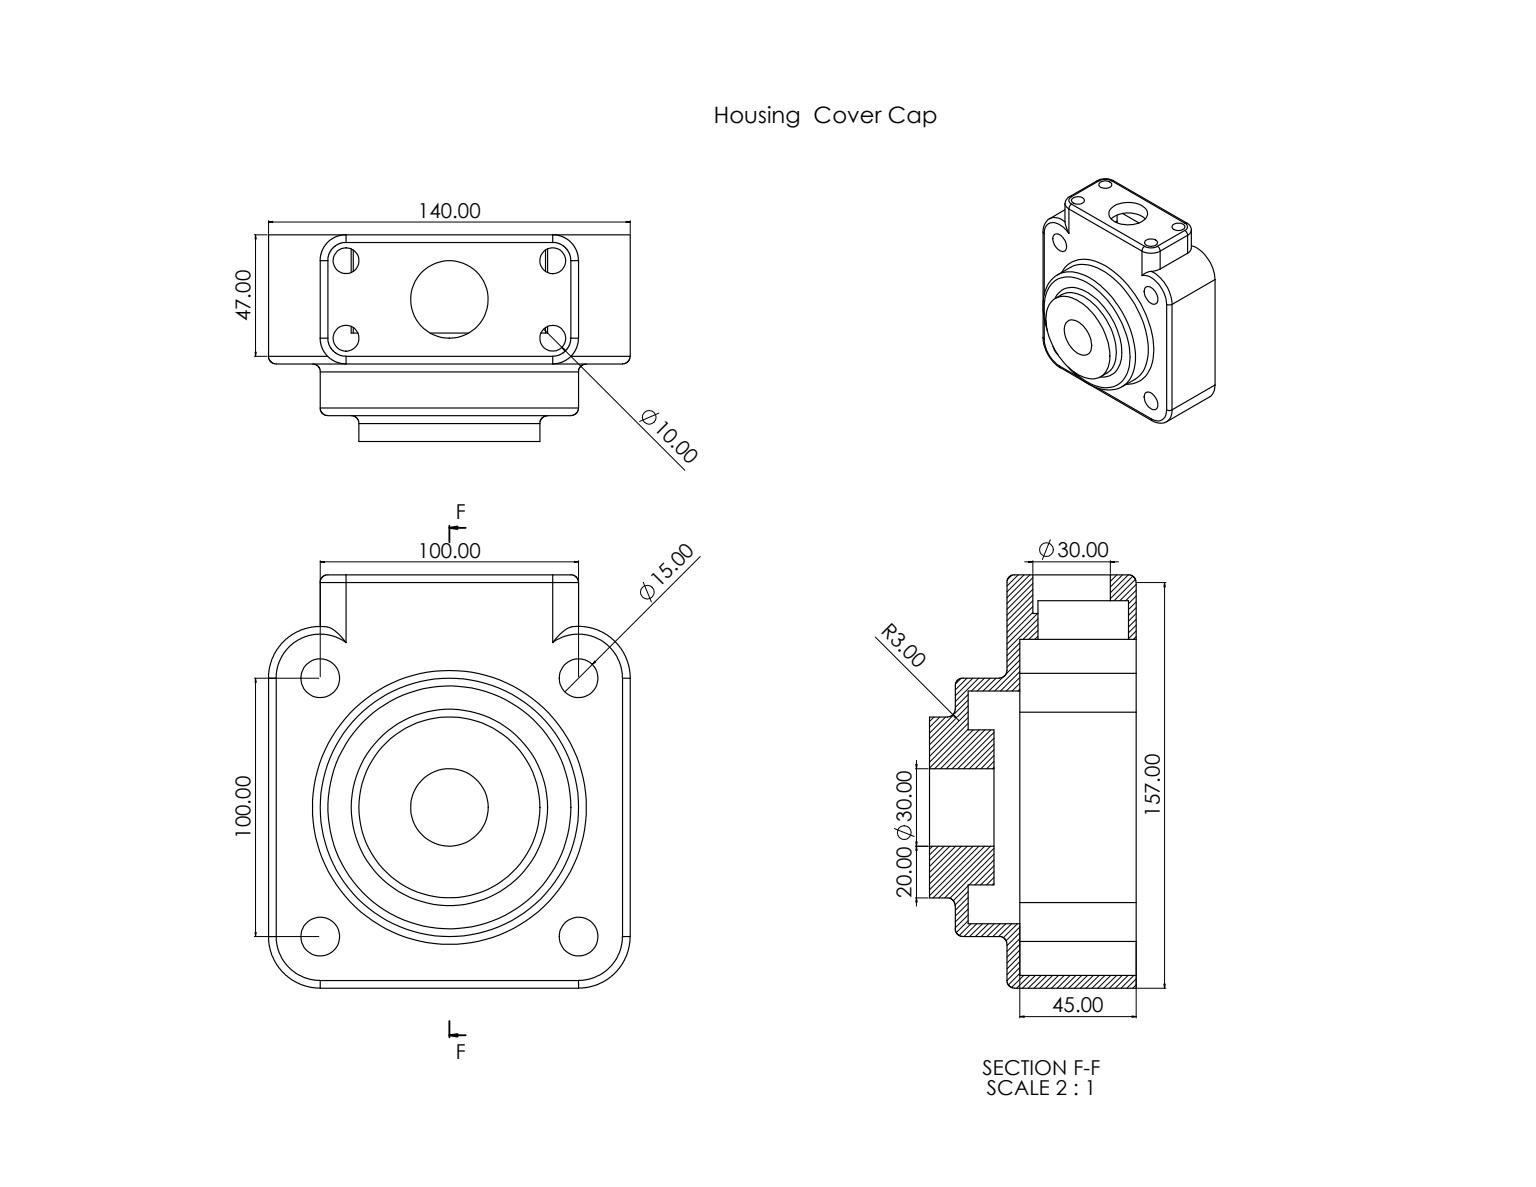
ISO-10303-21;
HEADER;
FILE_DESCRIPTION (('STEP AP214'),
    '1' );
FILE_NAME ('Housing  Cover Cap.step',
    '2026-10-18T20:16:25',
    ( '' ),
    ( '' ),
    'SwSTEP 2.0',
    'SolidWorks 2025',
    '' );
FILE_SCHEMA (( 'AUTOMOTIVE_DESIGN' ));
ENDSEC;

DATA;
#3=CARTESIAN_POINT ( 'NONE',  ( 37.16608720827707657, 51.86186943028246787, 12.49999999999999112 ) ) ;
#18=VERTEX_POINT ( 'NONE', #24496 ) ;
#21=CARTESIAN_POINT ( 'NONE',  ( -49.99999999999955236, -4.926614671774132148E-13, 82.49999999999998579 ) ) ;
#23=LINE ( 'NONE', #9535, #4037 ) ;
#27=ADVANCED_FACE ( 'NONE', ( #781 ), #12350, .T. ) ;
#31=DIRECTION ( 'NONE',  ( 0.000000000000000000, 0.000000000000000000, 1.000000000000000000 ) ) ;
#50=AXIS2_PLACEMENT_3D ( 'NONE', #18602, #5013, #4398 ) ;
#93=ORIENTED_EDGE ( 'NONE', *, *, #3486, .F. ) ;
#114=CARTESIAN_POINT ( 'NONE',  ( 57.49999999999998579, -50.00000000000000000, 97.07879600563551037 ) ) ;
#119=VERTEX_POINT ( 'NONE', #15443 ) ;
#124=AXIS2_PLACEMENT_3D ( 'NONE', #18042, #3695, #8540 ) ;
#129=ORIENTED_EDGE ( 'NONE', *, *, #25599, .F. ) ;
#146=ORIENTED_EDGE ( 'NONE', *, *, #2958, .F. ) ;
#148=CARTESIAN_POINT ( 'NONE',  ( -37.16608720827707657, -65.00000000000000000, 57.49999999999999289 ) ) ;
#164=DIRECTION ( 'NONE',  ( 1.000000000000000000, -0.000000000000000000, 0.000000000000000000 ) ) ;
#185=ORIENTED_EDGE ( 'NONE', *, *, #19570, .F. ) ;
#196=CARTESIAN_POINT ( 'NONE',  ( 39.99999999999998579, 87.00000000000001421, 12.49999999999999112 ) ) ;
#201=EDGE_CURVE ( 'NONE', #20672, #10252, #28885, .T. ) ;
#207=EDGE_CURVE ( 'NONE', #23407, #26039, #29815, .T. ) ;
#210=EDGE_CURVE ( 'NONE', #17431, #24948, #5944, .T. ) ;
#218=ORIENTED_EDGE ( 'NONE', *, *, #11268, .F. ) ;
#219=CARTESIAN_POINT ( 'NONE',  ( 50.00000000000045475, -4.865382331816764069E-13, 79.49999999999998579 ) ) ;
#228=VERTEX_POINT ( 'NONE', #15599 ) ;
#232=EDGE_CURVE ( 'NONE', #24670, #7391, #17304, .T. ) ;
#234=ADVANCED_FACE ( 'NONE', ( #15282 ), #1429, .T. ) ;
#238=EDGE_CURVE ( 'NONE', #14629, #10409, #29758, .T. ) ;
#241=EDGE_LOOP ( 'NONE', ( #4483, #26412, #12849, #13561 ) ) ;
#243=ADVANCED_FACE ( 'NONE', ( #23525 ), #20886, .F. ) ;
#270=ORIENTED_EDGE ( 'NONE', *, *, #22948, .T. ) ;
#284=ORIENTED_EDGE ( 'NONE', *, *, #16662, .T. ) ;
#291=PLANE ( 'NONE',  #12367 ) ;
#300=ORIENTED_EDGE ( 'NONE', *, *, #15085, .F. ) ;
#325=DIRECTION ( 'NONE',  ( 1.000000000000000000, 0.000000000000000000, 0.000000000000000000 ) ) ;
#327=DIRECTION ( 'NONE',  ( 1.000000000000000000, 0.000000000000000000, 0.000000000000000000 ) ) ;
#330=DIRECTION ( 'NONE',  ( 0.000000000000000000, 1.000000000000000000, -0.000000000000000000 ) ) ;
#340=CIRCLE ( 'NONE', #26766, 5.000000000000004441 ) ;
#346=VERTEX_POINT ( 'NONE', #26975 ) ;
#353=VERTEX_POINT ( 'NONE', #24142 ) ;
#375=DIRECTION ( 'NONE',  ( 0.000000000000000000, 0.000000000000000000, -1.000000000000000000 ) ) ;
#380=DIRECTION ( 'NONE',  ( 0.000000000000000000, 0.000000000000000000, 1.000000000000000000 ) ) ;
#381=EDGE_CURVE ( 'NONE', #9423, #9573, #2631, .T. ) ;
#390=CARTESIAN_POINT ( 'NONE',  ( 4.510281037539698445E-13, -4.926614671774132148E-13, 82.49999999999998579 ) ) ;
#392=ORIENTED_EDGE ( 'NONE', *, *, #26901, .T. ) ;
#395=EDGE_CURVE ( 'NONE', #119, #19467, #10261, .T. ) ;
#405=ORIENTED_EDGE ( 'NONE', *, *, #28102, .T. ) ;
#406=LINE ( 'NONE', #14743, #17330 ) ;
#412=EDGE_CURVE ( 'NONE', #8092, #2167, #25816, .T. ) ;
#422=ADVANCED_FACE ( 'NONE', ( #3565 ), #20954, .T. ) ;
#433=( LENGTH_UNIT ( ) NAMED_UNIT ( * ) SI_UNIT ( .MILLI., .METRE. ) );
#436=EDGE_CURVE ( 'NONE', #11277, #20672, #12935, .T. ) ;
#445=CARTESIAN_POINT ( 'NONE',  ( -50.00000000000000000, -50.00000000000000000, 97.07879600563551037 ) ) ;
#482=EDGE_CURVE ( 'NONE', #4513, #14016, #6055, .T. ) ;
#483=ADVANCED_FACE ( 'NONE', ( #14572 ), #23758, .T. ) ;
#498=VERTEX_POINT ( 'NONE', #7558 ) ;
#509=VERTEX_POINT ( 'NONE', #21581 ) ;
#528=FACE_OUTER_BOUND ( 'NONE', #3439, .T. ) ;
#532=AXIS2_PLACEMENT_3D ( 'NONE', #23516, #28832, #23662 ) ;
#535=EDGE_LOOP ( 'NONE', ( #1765, #22234, #5440, #4015 ) ) ;
#552=ADVANCED_FACE ( 'NONE', ( #7235 ), #23923, .F. ) ;
#569=ORIENTED_EDGE ( 'NONE', *, *, #16803, .T. ) ;
#628=CARTESIAN_POINT ( 'NONE',  ( -38.00000000000000711, 80.00000000000000000, 47.91742430504431383 ) ) ;
#634=AXIS2_PLACEMENT_3D ( 'NONE', #23126, #15969, #13490 ) ;
#640=DIRECTION ( 'NONE',  ( 1.000000000000000000, 0.000000000000000000, 4.565061778886335400E-17 ) ) ;
#648=CARTESIAN_POINT ( 'NONE',  ( -37.16608720827707657, 51.86186943028246787, 57.49999999999999289 ) ) ;
#655=AXIS2_PLACEMENT_3D ( 'NONE', #16975, #24609, #740 ) ;
#667=EDGE_LOOP ( 'NONE', ( #2923, #26532 ) ) ;
#671=DIRECTION ( 'NONE',  ( 0.000000000000000000, 0.000000000000000000, -1.000000000000000000 ) ) ;
#682=LINE ( 'NONE', #19245, #27844 ) ;
#702=FACE_OUTER_BOUND ( 'NONE', #5275, .T. ) ;
#707=PLANE ( 'NONE',  #25288 ) ;
#712=DIRECTION ( 'NONE',  ( 0.000000000000000000, -0.000000000000000000, 1.000000000000000000 ) ) ;
#719=DIRECTION ( 'NONE',  ( -1.000000000000000000, 1.224646799147308341E-16, 0.000000000000000000 ) ) ;
#731=PLANE ( 'NONE',  #2299 ) ;
#737=ORIENTED_EDGE ( 'NONE', *, *, #28020, .T. ) ;
#740=DIRECTION ( 'NONE',  ( 0.000000000000000000, 0.000000000000000000, -1.000000000000000000 ) ) ;
#747=ORIENTED_EDGE ( 'NONE', *, *, #23123, .T. ) ;
#754=AXIS2_PLACEMENT_3D ( 'NONE', #13903, #20910, #9218 ) ;
#756=DIRECTION ( 'NONE',  ( 0.000000000000000000, 0.000000000000000000, -1.000000000000000000 ) ) ;
#761=CARTESIAN_POINT ( 'NONE',  ( -67.00000000000000000, -50.00000000000000000, 62.49999999999999289 ) ) ;
#779=CARTESIAN_POINT ( 'NONE',  ( 49.75074519532149964, 69.99854282640310998, 54.74199497519533253 ) ) ;
#781=FACE_OUTER_BOUND ( 'NONE', #26889, .T. ) ;
#794=CARTESIAN_POINT ( 'NONE',  ( 46.83962869229247872, 69.75107682583961832, 59.80789731659786668 ) ) ;
#816=EDGE_LOOP ( 'NONE', ( #10122, #28506 ) ) ;
#817=ORIENTED_EDGE ( 'NONE', *, *, #19707, .F. ) ;
#822=CIRCLE ( 'NONE', #25229, 3.000000000000002665 ) ;
#833=CARTESIAN_POINT ( 'NONE',  ( -7.075845757273814415E-16, 65.00000000000000000, 15.49999999999998757 ) ) ;
#839=VECTOR ( 'NONE', #15202, 1000.000000000000000 ) ;
#847=ORIENTED_EDGE ( 'NONE', *, *, #7863, .T. ) ;
#854=DIRECTION ( 'NONE',  ( 1.000000000000000000, 0.000000000000000000, 0.000000000000000000 ) ) ;
#865=EDGE_CURVE ( 'NONE', #4126, #15180, #12302, .T. ) ;
#867=VECTOR ( 'NONE', #15137, 1000.000000000000000 ) ;
#869=DIRECTION ( 'NONE',  ( 0.000000000000000000, -0.000000000000000000, 1.000000000000000000 ) ) ;
#872=ORIENTED_EDGE ( 'NONE', *, *, #18796, .T. ) ;
#886=VERTEX_POINT ( 'NONE', #23419 ) ;
#921=ORIENTED_EDGE ( 'NONE', *, *, #28797, .F. ) ;
#932=LINE ( 'NONE', #24944, #23092 ) ;
#938=DIRECTION ( 'NONE',  ( -1.000000000000000000, 0.000000000000000000, 0.000000000000000000 ) ) ;
#941=AXIS2_PLACEMENT_3D ( 'NONE', #27026, #2189, #4376 ) ;
#945=DIRECTION ( 'NONE',  ( -1.000000000000000000, 0.000000000000000000, 0.000000000000000000 ) ) ;
#962=DIRECTION ( 'NONE',  ( 1.000000000000000000, 0.000000000000000000, 0.000000000000000000 ) ) ;
#963=VECTOR ( 'NONE', #30345, 1000.000000000000000 ) ;
#977=VERTEX_POINT ( 'NONE', #7367 ) ;
#980=CARTESIAN_POINT ( 'NONE',  ( 37.99999999999999289, 80.00000000000000000, 0.000000000000000000 ) ) ;
#987=ORIENTED_EDGE ( 'NONE', *, *, #11268, .T. ) ;
#996=DIRECTION ( 'NONE',  ( -1.000000000000000000, 0.000000000000000000, 0.000000000000000000 ) ) ;
#997=LINE ( 'NONE', #10507, #28045 ) ;
#1008=DIRECTION ( 'NONE',  ( 0.000000000000000000, 1.000000000000000000, -0.000000000000000000 ) ) ;
#1016=ORIENTED_EDGE ( 'NONE', *, *, #28061, .F. ) ;
#1019=LINE ( 'NONE', #10529, #11195 ) ;
#1024=LINE ( 'NONE', #9918, #9861 ) ;
#1030=CARTESIAN_POINT ( 'NONE',  ( 39.99999999999998579, 90.00000000000001421, 22.49999999999999289 ) ) ;
#1034=CARTESIAN_POINT ( 'NONE',  ( 39.99999999999998579, 90.00000000000001421, 52.49999999999999289 ) ) ;
#1043=CARTESIAN_POINT ( 'NONE',  ( -34.99999999999933920, 0.000000000000000000, 92.49999999999998579 ) ) ;
#1061=TOROIDAL_SURFACE ( 'NONE', #28508, 47.00000000000000000, 3.000000000000000000 ) ;
#1077=EDGE_LOOP ( 'NONE', ( #13664, #21788, #28119, #28909 ) ) ;
#1085=FACE_OUTER_BOUND ( 'NONE', #15743, .T. ) ;
#1094=VECTOR ( 'NONE', #9657, 1000.000000000000000 ) ;
#1114=DIRECTION ( 'NONE',  ( -1.000000000000000000, 0.000000000000000000, 0.000000000000000000 ) ) ;
#1118=ORIENTED_EDGE ( 'NONE', *, *, #29975, .T. ) ;
#1120=CARTESIAN_POINT ( 'NONE',  ( -41.02681369128806210, 65.11862996399604242, 62.46341648537969604 ) ) ;
#1132=AXIS2_PLACEMENT_3D ( 'NONE', #11394, #25726, #23672 ) ;
#1133=ORIENTED_EDGE ( 'NONE', *, *, #18687, .F. ) ;
#1151=AXIS2_PLACEMENT_3D ( 'NONE', #10819, #20330, #13767 ) ;
#1157=DIRECTION ( 'NONE',  ( -1.000000000000000000, 0.000000000000000000, 0.000000000000000000 ) ) ;
#1160=ORIENTED_EDGE ( 'NONE', *, *, #25599, .T. ) ;
#1161=DIRECTION ( 'NONE',  ( -0.000000000000000000, -0.000000000000000000, 1.000000000000000000 ) ) ;
#1189=CYLINDRICAL_SURFACE ( 'NONE', #21253, 10.00000000000000178 ) ;
#1215=ADVANCED_FACE ( 'NONE', ( #8102 ), #291, .T. ) ;
#1221=FACE_BOUND ( 'NONE', #816, .T. ) ;
#1222=VERTEX_POINT ( 'NONE', #12775 ) ;
#1225=ORIENTED_EDGE ( 'NONE', *, *, #15509, .T. ) ;
#1238=CARTESIAN_POINT ( 'NONE',  ( 0.000000000000000000, 0.000000000000000000, 82.49999999999998579 ) ) ;
#1243=CARTESIAN_POINT ( 'NONE',  ( 49.45745851869548204, 69.99439104891119712, 19.18218888609259665 ) ) ;
#1244=FACE_OUTER_BOUND ( 'NONE', #9042, .T. ) ;
#1252=LINE ( 'NONE', #3268, #8766 ) ;
#1257=ORIENTED_EDGE ( 'NONE', *, *, #26177, .F. ) ;
#1293=DIRECTION ( 'NONE',  ( 0.000000000000000000, -0.000000000000000000, -1.000000000000000000 ) ) ;
#1295=ORIENTED_EDGE ( 'NONE', *, *, #22144, .F. ) ;
#1301=AXIS2_PLACEMENT_3D ( 'NONE', #4447, #20953, #23150 ) ;
#1316=LINE ( 'NONE', #30013, #9536 ) ;
#1327=EDGE_CURVE ( 'NONE', #25485, #25063, #15100, .T. ) ;
#1349=LINE ( 'NONE', #8378, #16772 ) ;
#1356=DIRECTION ( 'NONE',  ( -1.000000000000000000, 0.000000000000000000, 0.000000000000000000 ) ) ;
#1365=EDGE_LOOP ( 'NONE', ( #17122, #18661, #20473, #30492 ) ) ;
#1369=AXIS2_PLACEMENT_3D ( 'NONE', #4710, #21541, #14681 ) ;
#1372=ORIENTED_EDGE ( 'NONE', *, *, #17855, .F. ) ;
#1376=VECTOR ( 'NONE', #15752, 1000.000000000000000 ) ;
#1403=CARTESIAN_POINT ( 'NONE',  ( 49.99999999999998579, 70.00000000000001421, 21.82070150977413903 ) ) ;
#1407=DIRECTION ( 'NONE',  ( 0.000000000000000000, 0.000000000000000000, 1.000000000000000000 ) ) ;
#1415=ORIENTED_EDGE ( 'NONE', *, *, #25806, .F. ) ;
#1418=EDGE_LOOP ( 'NONE', ( #23104, #19972, #12540, #30228 ) ) ;
#1423=ORIENTED_EDGE ( 'NONE', *, *, #5801, .F. ) ;
#1429=CYLINDRICAL_SURFACE ( 'NONE', #20294, 20.00000000000000355 ) ;
#1433=ORIENTED_EDGE ( 'NONE', *, *, #18979, .T. ) ;
#1440=FACE_BOUND ( 'NONE', #28403, .T. ) ;
#1442=CARTESIAN_POINT ( 'NONE',  ( 66.99999999999998579, 50.00000000000000000, 59.49999999999999289 ) ) ;
#1463=CARTESIAN_POINT ( 'NONE',  ( 66.99999999999998579, 50.00000000000000000, 62.49999999999999289 ) ) ;
#1468=AXIS2_PLACEMENT_3D ( 'NONE', #28004, #20963, #1806 ) ;
#1479=CARTESIAN_POINT ( 'NONE',  ( 49.99999999999998579, 50.00000000000000000, 12.49999999999999112 ) ) ;
#1515=CARTESIAN_POINT ( 'NONE',  ( 4.510281037539698445E-13, -4.926614671774132148E-13, 65.49999999999998579 ) ) ;
#1524=EDGE_CURVE ( 'NONE', #8240, #3050, #30833, .T. ) ;
#1528=CARTESIAN_POINT ( 'NONE',  ( -40.00000000000000000, 90.00000000000001421, 12.49999999999999112 ) ) ;
#1536=FACE_OUTER_BOUND ( 'NONE', #20558, .T. ) ;
#1548=CARTESIAN_POINT ( 'NONE',  ( 47.38379984956800683, 69.82936349420988620, 15.74781942413362401 ) ) ;
#1551=AXIS2_PLACEMENT_3D ( 'NONE', #27356, #5980, #30295 ) ;
#1572=EDGE_CURVE ( 'NONE', #27348, #886, #4923, .T. ) ;
#1577=ORIENTED_EDGE ( 'NONE', *, *, #1998, .F. ) ;
#1588=ORIENTED_EDGE ( 'NONE', *, *, #27343, .F. ) ;
#1589=CARTESIAN_POINT ( 'NONE',  ( 39.99999999999998579, 80.00000000000001421, 27.49999999999998934 ) ) ;
#1598=LINE ( 'NONE', #25900, #7425 ) ;
#1608=EDGE_CURVE ( 'NONE', #30496, #8380, #2142, .T. ) ;
#1616=CARTESIAN_POINT ( 'NONE',  ( 47.14142842854284510, 69.79466010243311302, 59.49999999999998579 ) ) ;
#1628=CARTESIAN_POINT ( 'NONE',  ( -38.00000000000000711, 65.00000000000000000, 50.49999999999998579 ) ) ;
#1646=FACE_OUTER_BOUND ( 'NONE', #22033, .T. ) ;
#1653=CARTESIAN_POINT ( 'NONE',  ( -47.82582523423074861, 69.88269270952190482, 16.26542374043941308 ) ) ;
#1663=DIRECTION ( 'NONE',  ( -1.000000000000000000, 0.000000000000000000, 0.000000000000000000 ) ) ;
#1684=VECTOR ( 'NONE', #5109, 1000.000000000000000 ) ;
#1688=VECTOR ( 'NONE', #24091, 1000.000000000000000 ) ;
#1696=ORIENTED_EDGE ( 'NONE', *, *, #28797, .T. ) ;
#1705=CIRCLE ( 'NONE', #23109, 3.000000000000002665 ) ;
#1714=CARTESIAN_POINT ( 'NONE',  ( -64.99999999999998579, -36.86186943028246787, 97.07879600563551037 ) ) ;
#1726=EDGE_LOOP ( 'NONE', ( #5104, #22705, #1867, #28955 ) ) ;
#1729=CARTESIAN_POINT ( 'NONE',  ( 39.99999999999998579, 90.00000000000001421, 59.49999999999999289 ) ) ;
#1736=LINE ( 'NONE', #23090, #25376 ) ;
#1747=ORIENTED_EDGE ( 'NONE', *, *, #14163, .F. ) ;
#1765=ORIENTED_EDGE ( 'NONE', *, *, #23091, .F. ) ;
#1771=ORIENTED_EDGE ( 'NONE', *, *, #28051, .F. ) ;
#1796=AXIS2_PLACEMENT_3D ( 'NONE', #16884, #14215, #26081 ) ;
#1799=FACE_OUTER_BOUND ( 'NONE', #1077, .T. ) ;
#1804=DIRECTION ( 'NONE',  ( 0.000000000000000000, 0.000000000000000000, 1.000000000000000000 ) ) ;
#1806=DIRECTION ( 'NONE',  ( 1.000000000000000000, 0.000000000000000000, 0.000000000000000000 ) ) ;
#1811=ORIENTED_EDGE ( 'NONE', *, *, #210, .F. ) ;
#1815=CARTESIAN_POINT ( 'NONE',  ( 53.00000000000045475, -4.861708391419322267E-13, 65.49999999999998579 ) ) ;
#1836=( NAMED_UNIT ( * ) PLANE_ANGLE_UNIT ( ) SI_UNIT ( $, .RADIAN. ) );
#1837=DIRECTION ( 'NONE',  ( -0.000000000000000000, 1.000000000000000000, -0.000000000000000000 ) ) ;
#1838=CARTESIAN_POINT ( 'NONE',  ( 39.99999999999998579, 80.00000000000001421, 17.49999999999999645 ) ) ;
#1841=AXIS2_PLACEMENT_3D ( 'NONE', #15376, #12910, #15536 ) ;
#1849=ORIENTED_EDGE ( 'NONE', *, *, #22349, .F. ) ;
#1857=DIRECTION ( 'NONE',  ( -0.000000000000000000, 1.000000000000000000, 0.000000000000000000 ) ) ;
#1861=ORIENTED_EDGE ( 'NONE', *, *, #16788, .T. ) ;
#1867=ORIENTED_EDGE ( 'NONE', *, *, #2489, .T. ) ;
#1868=AXIS2_PLACEMENT_3D ( 'NONE', #21433, #375, #22045 ) ;
#1892=AXIS2_PLACEMENT_3D ( 'NONE', #14281, #24110, #26306 ) ;
#1915=FACE_OUTER_BOUND ( 'NONE', #241, .T. ) ;
#1933=CARTESIAN_POINT ( 'NONE',  ( -15.00000000000004086, 1.571475800653548713E-14, 67.49999999999997158 ) ) ;
#1947=ADVANCED_FACE ( 'NONE', ( #3996 ), #10402, .F. ) ;
#1972=ADVANCED_FACE ( 'NONE', ( #14100 ), #16903, .F. ) ;
#1998=EDGE_CURVE ( 'NONE', #7862, #25485, #16458, .T. ) ;
#2013=ORIENTED_EDGE ( 'NONE', *, *, #27648, .F. ) ;
#2030=ORIENTED_EDGE ( 'NONE', *, *, #27366, .F. ) ;
#2037=DIRECTION ( 'NONE',  ( -1.000000000000000000, -0.000000000000000000, -0.000000000000000000 ) ) ;
#2056=ORIENTED_EDGE ( 'NONE', *, *, #20964, .F. ) ;
#2080=LINE ( 'NONE', #28140, #25328 ) ;
#2081=ORIENTED_EDGE ( 'NONE', *, *, #17855, .T. ) ;
#2085=CYLINDRICAL_SURFACE ( 'NONE', #8887, 29.99999999999928946 ) ;
#2088=CARTESIAN_POINT ( 'NONE',  ( 49.99999999999998579, 50.00000000000000000, 12.49999999999999112 ) ) ;
#2129=CARTESIAN_POINT ( 'NONE',  ( -57.50000000000001421, -50.00000000000000000, 12.49999999999999112 ) ) ;
#2133=( NAMED_UNIT ( * ) SI_UNIT ( $, .STERADIAN. ) SOLID_ANGLE_UNIT ( ) );
#2134=EDGE_CURVE ( 'NONE', #12801, #20802, #16920, .T. ) ;
#2138=ADVANCED_FACE ( 'NONE', ( #20141 ), #26435, .F. ) ;
#2142=LINE ( 'NONE', #2458, #29836 ) ;
#2150=CIRCLE ( 'NONE', #25556, 3.000000000000002665 ) ;
#2152=ADVANCED_FACE ( 'NONE', ( #24081 ), #22326, .T. ) ;
#2158=LINE ( 'NONE', #20876, #18238 ) ;
#2162=ORIENTED_EDGE ( 'NONE', *, *, #238, .F. ) ;
#2164=DIRECTION ( 'NONE',  ( 1.000000000000000000, 0.000000000000000000, 0.000000000000000000 ) ) ;
#2167=VERTEX_POINT ( 'NONE', #23767 ) ;
#2174=LINE ( 'NONE', #21178, #5076 ) ;
#2179=DIRECTION ( 'NONE',  ( -1.000000000000000000, 0.000000000000000000, 0.000000000000000000 ) ) ;
#2189=DIRECTION ( 'NONE',  ( 0.000000000000000000, 0.000000000000000000, -1.000000000000000000 ) ) ;
#2190=AXIS2_PLACEMENT_3D ( 'NONE', #7061, #2386, #6916 ) ;
#2198=ORIENTED_EDGE ( 'NONE', *, *, #12967, .F. ) ;
#2208=VECTOR ( 'NONE', #8117, 1000.000000000000000 ) ;
#2243=DIRECTION ( 'NONE',  ( 0.000000000000000000, 0.000000000000000000, 1.000000000000000000 ) ) ;
#2283=CIRCLE ( 'NONE', #19724, 15.00000000000000000 ) ;
#2299=AXIS2_PLACEMENT_3D ( 'NONE', #17276, #15551, #26809 ) ;
#2311=ORIENTED_EDGE ( 'NONE', *, *, #22140, .T. ) ;
#2313=VECTOR ( 'NONE', #14202, 1000.000000000000000 ) ;
#2317=DIRECTION ( 'NONE',  ( -0.000000000000000000, 1.000000000000000000, -0.000000000000000000 ) ) ;
#2324=ORIENTED_EDGE ( 'NONE', *, *, #18426, .T. ) ;
#2331=EDGE_LOOP ( 'NONE', ( #12248, #847, #22485, #24740 ) ) ;
#2373=ORIENTED_EDGE ( 'NONE', *, *, #8208, .T. ) ;
#2375=DIRECTION ( 'NONE',  ( -0.000000000000000000, -1.000000000000000000, -0.000000000000000000 ) ) ;
#2386=DIRECTION ( 'NONE',  ( 0.000000000000000000, 0.000000000000000000, 1.000000000000000000 ) ) ;
#2391=VECTOR ( 'NONE', #9153, 1000.000000000000000 ) ;
#2396=ORIENTED_EDGE ( 'NONE', *, *, #5540, .F. ) ;
#2399=ORIENTED_EDGE ( 'NONE', *, *, #24487, .T. ) ;
#2433=CIRCLE ( 'NONE', #26264, 29.99999999999928946 ) ;
#2449=CARTESIAN_POINT ( 'NONE',  ( 49.99999999999998579, -70.00000000000000000, 59.49999999999999289 ) ) ;
#2458=CARTESIAN_POINT ( 'NONE',  ( -52.16608720827707657, 36.86186943028246787, 97.07879600563551037 ) ) ;
#2479=ORIENTED_EDGE ( 'NONE', *, *, #16053, .F. ) ;
#2485=DIRECTION ( 'NONE',  ( -0.000000000000000000, -0.000000000000000000, 1.000000000000000000 ) ) ;
#2489=EDGE_CURVE ( 'NONE', #12801, #14860, #822, .T. ) ;
#2493=CARTESIAN_POINT ( 'NONE',  ( -34.99999999999933920, 0.000000000000000000, 92.49999999999998579 ) ) ;
#2498=EDGE_CURVE ( 'NONE', #28591, #119, #22243, .T. ) ;
#2520=ORIENTED_EDGE ( 'NONE', *, *, #6743, .F. ) ;
#2524=DIRECTION ( 'NONE',  ( 0.000000000000000000, 0.000000000000000000, 1.000000000000000000 ) ) ;
#2549=AXIS2_PLACEMENT_3D ( 'NONE', #12742, #10401, #25362 ) ;
#2550=DIRECTION ( 'NONE',  ( 1.000000000000000000, -0.000000000000000000, -0.000000000000000000 ) ) ;
#2558=ORIENTED_EDGE ( 'NONE', *, *, #18946, .F. ) ;
#2563=ADVANCED_FACE ( 'NONE', ( #12523 ), #16885, .F. ) ;
#2570=CARTESIAN_POINT ( 'NONE',  ( -50.00000000000000000, -50.00000000000000000, 97.07879600563551037 ) ) ;
#2571=VERTEX_POINT ( 'NONE', #18926 ) ;
#2574=CARTESIAN_POINT ( 'NONE',  ( 37.99999999999999289, 80.00000000000000000, 50.49999999999998579 ) ) ;
#2575=DIRECTION ( 'NONE',  ( 0.000000000000000000, 0.000000000000000000, 1.000000000000000000 ) ) ;
#2577=CARTESIAN_POINT ( 'NONE',  ( -40.00000000000002842, 80.00000000000001421, 22.49999999999983302 ) ) ;
#2583=DIRECTION ( 'NONE',  ( 0.000000000000000000, 0.000000000000000000, -1.000000000000000000 ) ) ;
#2600=ORIENTED_EDGE ( 'NONE', *, *, #27155, .F. ) ;
#2615=CARTESIAN_POINT ( 'NONE',  ( -50.00000000000000000, 70.00000000000000000, 52.49999999999999289 ) ) ;
#2620=ORIENTED_EDGE ( 'NONE', *, *, #14985, .F. ) ;
#2627=VERTEX_POINT ( 'NONE', #26083 ) ;
#2631=LINE ( 'NONE', #2790, #8152 ) ;
#2646=DIRECTION ( 'NONE',  ( -1.000000000000000000, 0.000000000000000000, 0.000000000000000000 ) ) ;
#2652=DIRECTION ( 'NONE',  ( -1.000000000000000000, 0.000000000000000000, 0.000000000000000000 ) ) ;
#2669=CARTESIAN_POINT ( 'NONE',  ( 47.14142842854284510, 69.79466010243311302, 59.49999999999998579 ) ) ;
#2683=EDGE_CURVE ( 'NONE', #27986, #27603, #13292, .T. ) ;
#2694=ORIENTED_EDGE ( 'NONE', *, *, #22140, .F. ) ;
#2695=LINE ( 'NONE', #14693, #30620 ) ;
#2707=ORIENTED_EDGE ( 'NONE', *, *, #10964, .F. ) ;
#2708=ORIENTED_EDGE ( 'NONE', *, *, #16097, .T. ) ;
#2727=DIRECTION ( 'NONE',  ( 0.000000000000000000, 0.000000000000000000, -1.000000000000000000 ) ) ;
#2729=ADVANCED_FACE ( 'NONE', ( #3302 ), #29195, .T. ) ;
#2731=DIRECTION ( 'NONE',  ( -1.000000000000000000, 0.000000000000000000, 0.000000000000000000 ) ) ;
#2738=FACE_OUTER_BOUND ( 'NONE', #21954, .T. ) ;
#2744=FACE_OUTER_BOUND ( 'NONE', #10004, .T. ) ;
#2767=ORIENTED_EDGE ( 'NONE', *, *, #20964, .T. ) ;
#2780=ORIENTED_EDGE ( 'NONE', *, *, #26439, .F. ) ;
#2783=AXIS2_PLACEMENT_3D ( 'NONE', #10452, #24794, #3433 ) ;
#2784=CARTESIAN_POINT ( 'NONE',  ( 39.99999999999998579, 90.00000000000001421, 52.49999999999999289 ) ) ;
#2790=CARTESIAN_POINT ( 'NONE',  ( 0.000000000000000000, 80.00000000000000000, 50.49999999999998579 ) ) ;
#2794=DIRECTION ( 'NONE',  ( -1.000000000000000000, 0.000000000000000000, 0.000000000000000000 ) ) ;
#2805=DIRECTION ( 'NONE',  ( 0.000000000000000000, 0.000000000000000000, -1.000000000000000000 ) ) ;
#2817=AXIS2_PLACEMENT_3D ( 'NONE', #30042, #10704, #17717 ) ;
#2828=FACE_OUTER_BOUND ( 'NONE', #10800, .T. ) ;
#2834=DIRECTION ( 'NONE',  ( -0.000000000000000000, -0.000000000000000000, -1.000000000000000000 ) ) ;
#2842=CARTESIAN_POINT ( 'NONE',  ( -15.00000000000004086, 1.571475800653548713E-14, 77.49999999999998579 ) ) ;
#2849=DIRECTION ( 'NONE',  ( -1.000000000000000000, 0.000000000000000000, 0.000000000000000000 ) ) ;
#2852=VERTEX_POINT ( 'NONE', #25230 ) ;
#2869=CARTESIAN_POINT ( 'NONE',  ( -40.00000000000002842, 80.00000000000001421, 22.49999999999983302 ) ) ;
#2876=CIRCLE ( 'NONE', #20316, 3.000000000000002665 ) ;
#2882=EDGE_CURVE ( 'NONE', #28303, #23905, #15716, .T. ) ;
#2883=ADVANCED_FACE ( 'NONE', ( #1536 ), #27117, .T. ) ;
#2896=ORIENTED_EDGE ( 'NONE', *, *, #7446, .T. ) ;
#2901=EDGE_CURVE ( 'NONE', #4862, #27728, #17918, .T. ) ;
#2923=ORIENTED_EDGE ( 'NONE', *, *, #7801, .F. ) ;
#2927=MANIFOLD_SOLID_BREP ( 'Cut-Extrude26', #14306 ) ;
#2928=VECTOR ( 'NONE', #11011, 1000.000000000000000 ) ;
#2951=AXIS2_PLACEMENT_3D ( 'NONE', #22402, #11018, #15373 ) ;
#2958=EDGE_CURVE ( 'NONE', #15108, #3647, #8323, .T. ) ;
#2969=ORIENTED_EDGE ( 'NONE', *, *, #16012, .F. ) ;
#2992=ADVANCED_FACE ( 'NONE', ( #7750 ), #26782, .F. ) ;
#2996=ORIENTED_EDGE ( 'NONE', *, *, #16605, .T. ) ;
#3003=CARTESIAN_POINT ( 'NONE',  ( -43.65325914805313801, 67.82531758386231502, 61.81444568807134488 ) ) ;
#3015=EDGE_LOOP ( 'NONE', ( #2324, #15455, #1577, #2558, #11670, #8360 ) ) ;
#3034=CARTESIAN_POINT ( 'NONE',  ( -50.00000000000000000, -50.00000000000000000, 59.49999999999999289 ) ) ;
#3038=VECTOR ( 'NONE', #12443, 1000.000000000000000 ) ;
#3042=CARTESIAN_POINT ( 'NONE',  ( 57.49999999999998579, -50.00000000000000000, 12.49999999999999112 ) ) ;
#3045=DIRECTION ( 'NONE',  ( -1.000000000000000000, 0.000000000000000000, 0.000000000000000000 ) ) ;
#3048=CARTESIAN_POINT ( 'NONE',  ( 49.99999999999998579, 90.00000000000001421, 22.49999999999999289 ) ) ;
#3050=VERTEX_POINT ( 'NONE', #4776 ) ;
#3056=CARTESIAN_POINT ( 'NONE',  ( -37.16608720827707657, -65.00000000000000000, 12.49999999999999112 ) ) ;
#3071=EDGE_LOOP ( 'NONE', ( #28632, #29334, #17079, #4765 ) ) ;
#3097=EDGE_CURVE ( 'NONE', #28559, #9226, #24111, .T. ) ;
#3099=ORIENTED_EDGE ( 'NONE', *, *, #24475, .T. ) ;
#3118=AXIS2_PLACEMENT_3D ( 'NONE', #7454, #26318, #14463 ) ;
#3123=CARTESIAN_POINT ( 'NONE',  ( -38.00000000000000000, 65.00000000000000000, -7.533656238527846826E-15 ) ) ;
#3127=DIRECTION ( 'NONE',  ( -1.000000000000000000, 0.000000000000000000, 0.000000000000000000 ) ) ;
#3132=ORIENTED_EDGE ( 'NONE', *, *, #10484, .F. ) ;
#3141=CARTESIAN_POINT ( 'NONE',  ( 39.99999999999998579, 80.00000000000001421, 52.49999999999999289 ) ) ;
#3167=DIRECTION ( 'NONE',  ( 0.000000000000000000, 0.000000000000000000, -1.000000000000000000 ) ) ;
#3200=CARTESIAN_POINT ( 'NONE',  ( -40.00000000000002842, 80.00000000000001421, 22.49999999999983302 ) ) ;
#3201=VECTOR ( 'NONE', #9905, 1000.000000000000000 ) ;
#3202=EDGE_LOOP ( 'NONE', ( #14173, #21790, #16560, #10752 ) ) ;
#3212=DIRECTION ( 'NONE',  ( 0.000000000000000000, -1.000000000000000000, 0.000000000000000000 ) ) ;
#3219=VECTOR ( 'NONE', #27139, 1000.000000000000000 ) ;
#3243=CARTESIAN_POINT ( 'NONE',  ( 0.000000000000000000, 80.00000000000000000, 50.49999999999998579 ) ) ;
#3250=EDGE_LOOP ( 'NONE', ( #27903, #20834, #20462, #18701 ) ) ;
#3253=DIRECTION ( 'NONE',  ( -0.000000000000000000, -1.000000000000000000, -0.000000000000000000 ) ) ;
#3264=CARTESIAN_POINT ( 'NONE',  ( 39.99999999999998579, 80.00000000000001421, 27.49999999999998934 ) ) ;
#3268=CARTESIAN_POINT ( 'NONE',  ( -37.16608720827707657, -36.86186943028246787, 57.49999999999999289 ) ) ;
#3276=ADVANCED_FACE ( 'NONE', ( #20816, #25355 ), #16144, .T. ) ;
#3282=EDGE_CURVE ( 'NONE', #24053, #16046, #17235, .T. ) ;
#3284=DIRECTION ( 'NONE',  ( 0.000000000000000000, 0.000000000000000000, -1.000000000000000000 ) ) ;
#3298=EDGE_CURVE ( 'NONE', #24948, #30496, #6763, .T. ) ;
#3299=CARTESIAN_POINT ( 'NONE',  ( -44.60412845616029642, 68.57966488780255077, 61.38406448208059629 ) ) ;
#3300=ADVANCED_FACE ( 'NONE', ( #1799 ), #10759, .T. ) ;
#3302=FACE_OUTER_BOUND ( 'NONE', #18032, .T. ) ;
#3313=LINE ( 'NONE', #980, #26168 ) ;
#3327=VECTOR ( 'NONE', #27041, 1000.000000000000000 ) ;
#3334=VECTOR ( 'NONE', #30663, 1000.000000000000000 ) ;
#3338=FACE_OUTER_BOUND ( 'NONE', #7004, .T. ) ;
#3355=CARTESIAN_POINT ( 'NONE',  ( 37.16608720827707657, 65.00000000000000000, 15.49999999999998579 ) ) ;
#3360=AXIS2_PLACEMENT_3D ( 'NONE', #18000, #24385, #10506 ) ;
#3376=CARTESIAN_POINT ( 'NONE',  ( -38.00000000000000000, 80.00000000000000000, 15.49999999999998579 ) ) ;
#3385=DIRECTION ( 'NONE',  ( 0.000000000000000000, 0.000000000000000000, -1.000000000000000000 ) ) ;
#3387=AXIS2_PLACEMENT_3D ( 'NONE', #21191, #7179, #21364 ) ;
#3399=ORIENTED_EDGE ( 'NONE', *, *, #6115, .T. ) ;
#3403=DIRECTION ( 'NONE',  ( 0.000000000000000000, 1.000000000000000000, -0.000000000000000000 ) ) ;
#3422=ORIENTED_EDGE ( 'NONE', *, *, #23671, .T. ) ;
#3427=DIRECTION ( 'NONE',  ( -0.000000000000000000, 1.000000000000000000, -0.000000000000000000 ) ) ;
#3433=DIRECTION ( 'NONE',  ( -1.000000000000000000, 0.000000000000000000, 0.000000000000000000 ) ) ;
#3439=EDGE_LOOP ( 'NONE', ( #6605, #15249, #21286, #2969 ) ) ;
#3442=AXIS2_PLACEMENT_3D ( 'NONE', #1815, #20675, #30495 ) ;
#3450=VECTOR ( 'NONE', #17861, 1000.000000000000000 ) ;
#3459=VECTOR ( 'NONE', #29508, 1000.000000000000000 ) ;
#3463=ORIENTED_EDGE ( 'NONE', *, *, #5222, .F. ) ;
#3470=EDGE_CURVE ( 'NONE', #20725, #4577, #2283, .T. ) ;
#3472=EDGE_CURVE ( 'NONE', #5139, #19648, #29859, .T. ) ;
#3486=EDGE_CURVE ( 'NONE', #15921, #14016, #18002, .T. ) ;
#3496=DIRECTION ( 'NONE',  ( 0.000000000000000000, 0.000000000000000000, -1.000000000000000000 ) ) ;
#3507=DIRECTION ( 'NONE',  ( -1.000000000000000000, 0.000000000000000000, 0.000000000000000000 ) ) ;
#3528=FACE_BOUND ( 'NONE', #12397, .T. ) ;
#3556=FACE_BOUND ( 'NONE', #28413, .T. ) ;
#3565=FACE_OUTER_BOUND ( 'NONE', #17971, .T. ) ;
#3567=CARTESIAN_POINT ( 'NONE',  ( -40.00000000000002842, 80.00000000000001421, 47.50000000000014921 ) ) ;
#3572=ADVANCED_BREP_SHAPE_REPRESENTATION ( '', ( #2927, #7396 ), #10404 ) ;
#3578=CARTESIAN_POINT ( 'NONE',  ( 43.00084836024851143, 68.73816704320454107, 12.95563330655122769 ) ) ;
#3579=DIRECTION ( 'NONE',  ( 0.000000000000000000, 0.000000000000000000, 1.000000000000000000 ) ) ;
#3594=CYLINDRICAL_SURFACE ( 'NONE', #29842, 5.000000000000004441 ) ;
#3599=DIRECTION ( 'NONE',  ( 0.000000000000000000, 0.000000000000000000, 1.000000000000000000 ) ) ;
#3601=APPLICATION_CONTEXT ( 'automotive_design' ) ;
#3605=ORIENTED_EDGE ( 'NONE', *, *, #27343, .T. ) ;
#3619=CARTESIAN_POINT ( 'NONE',  ( 39.99999999999998579, 80.00000000000001421, 57.49999999999998579 ) ) ;
#3630=ORIENTED_EDGE ( 'NONE', *, *, #14923, .T. ) ;
#3631=CARTESIAN_POINT ( 'NONE',  ( -40.00000000000002842, 80.00000000000001421, 22.49999999999983302 ) ) ;
#3635=CARTESIAN_POINT ( 'NONE',  ( 52.16608720827707657, -36.86186943028246787, 57.49999999999999289 ) ) ;
#3636=VERTEX_POINT ( 'NONE', #27122 ) ;
#3641=CYLINDRICAL_SURFACE ( 'NONE', #22791, 4.999999999999997335 ) ;
#3647=VERTEX_POINT ( 'NONE', #10736 ) ;
#3653=AXIS2_PLACEMENT_3D ( 'NONE', #26908, #17225, #5224 ) ;
#3661=EDGE_CURVE ( 'NONE', #25063, #23409, #21716, .T. ) ;
#3680=AXIS2_PLACEMENT_3D ( 'NONE', #27292, #1407, #18087 ) ;
#3688=CARTESIAN_POINT ( 'NONE',  ( -50.00000000000000000, 50.00000000000000000, 12.49999999999999112 ) ) ;
#3695=DIRECTION ( 'NONE',  ( 4.565061778886335400E-17, 0.000000000000000000, -1.000000000000000000 ) ) ;
#3703=CIRCLE ( 'NONE', #6670, 4.999999999999997335 ) ;
#3706=SHAPE_REPRESENTATION_RELATIONSHIP ( 'NONE' , 'NONE' ,  #13696, #3572 ) ;
#3722=CIRCLE ( 'NONE', #9186, 20.00000000000000355 ) ;
#3738=CARTESIAN_POINT ( 'NONE',  ( 46.67303262113644990, 69.72284517594248143, 15.04469359926350336 ) ) ;
#3739=DIRECTION ( 'NONE',  ( -1.000000000000000000, 0.000000000000000000, 0.000000000000000000 ) ) ;
#3742=DIRECTION ( 'NONE',  ( 0.000000000000000000, 0.000000000000000000, -1.000000000000000000 ) ) ;
#3746=DIRECTION ( 'NONE',  ( -0.000000000000000000, -0.000000000000000000, 1.000000000000000000 ) ) ;
#3757=DIRECTION ( 'NONE',  ( 6.938893903907227392E-16, 0.000000000000000000, 1.000000000000000000 ) ) ;
#3776=DIRECTION ( 'NONE',  ( 0.000000000000000000, 0.000000000000000000, -1.000000000000000000 ) ) ;
#3777=AXIS2_PLACEMENT_3D ( 'NONE', #6810, #28958, #5252 ) ;
#3809=ORIENTED_EDGE ( 'NONE', *, *, #14903, .F. ) ;
#3831=CARTESIAN_POINT ( 'NONE',  ( 64.99999999999998579, -36.86186943028246787, 97.07879600563551037 ) ) ;
#3837=DIRECTION ( 'NONE',  ( 0.000000000000000000, -0.000000000000000000, 1.000000000000000000 ) ) ;
#3848=CARTESIAN_POINT ( 'NONE',  ( 49.99999999999998579, -50.00000000000000000, 62.49999999999999289 ) ) ;
#3849=DIRECTION ( 'NONE',  ( 1.000000000000000000, 0.000000000000000000, 0.000000000000000000 ) ) ;
#3851=DIRECTION ( 'NONE',  ( -1.000000000000000000, 0.000000000000000000, 0.000000000000000000 ) ) ;
#3862=DIRECTION ( 'NONE',  ( 0.000000000000000000, -0.000000000000000000, 1.000000000000000000 ) ) ;
#3874=TOROIDAL_SURFACE ( 'NONE', #21779, 7.000000000000000000, 3.000000000000000000 ) ;
#3891=AXIS2_PLACEMENT_3D ( 'NONE', #13671, #11016, #25361 ) ;
#3894=CARTESIAN_POINT ( 'NONE',  ( 44.78385332603417623, 69.31632679361693761, 13.69377121817660914 ) ) ;
#3899=LINE ( 'NONE', #25099, #23576 ) ;
#3904=VERTEX_POINT ( 'NONE', #19594 ) ;
#3932=ORIENTED_EDGE ( 'NONE', *, *, #29834, .F. ) ;
#3944=ORIENTED_EDGE ( 'NONE', *, *, #395, .T. ) ;
#3953=CARTESIAN_POINT ( 'NONE',  ( -40.00000000000000000, 87.00000000000001421, 59.49999999999999289 ) ) ;
#3958=DIRECTION ( 'NONE',  ( -0.000000000000000000, 0.000000000000000000, 1.000000000000000000 ) ) ;
#3964=EDGE_LOOP ( 'NONE', ( #10725, #2520 ) ) ;
#3971=ORIENTED_EDGE ( 'NONE', *, *, #10885, .T. ) ;
#3972=CARTESIAN_POINT ( 'NONE',  ( -2.081668171172168513E-14, 75.00000000000001421, 37.49999999999999289 ) ) ;
#3978=ORIENTED_EDGE ( 'NONE', *, *, #412, .F. ) ;
#3986=TOROIDAL_SURFACE ( 'NONE', #25903, 17.00000000000000000, 3.000000000000000000 ) ;
#3996=FACE_OUTER_BOUND ( 'NONE', #27575, .T. ) ;
#4001=FACE_BOUND ( 'NONE', #25427, .T. ) ;
#4009=ORIENTED_EDGE ( 'NONE', *, *, #18946, .T. ) ;
#4010=ORIENTED_EDGE ( 'NONE', *, *, #6742, .T. ) ;
#4015=ORIENTED_EDGE ( 'NONE', *, *, #23131, .F. ) ;
#4017=DIRECTION ( 'NONE',  ( 0.000000000000000000, 1.000000000000000000, 0.000000000000000000 ) ) ;
#4018=ORIENTED_EDGE ( 'NONE', *, *, #15307, .F. ) ;
#4037=VECTOR ( 'NONE', #9389, 1000.000000000000000 ) ;
#4038=DIRECTION ( 'NONE',  ( -0.000000000000000000, -0.000000000000000000, -1.000000000000000000 ) ) ;
#4072=FACE_OUTER_BOUND ( 'NONE', #29918, .T. ) ;
#4083=ORIENTED_EDGE ( 'NONE', *, *, #3661, .T. ) ;
#4097=DIRECTION ( 'NONE',  ( -1.000000000000000000, 0.000000000000000000, -0.000000000000000000 ) ) ;
#4099=DIRECTION ( 'NONE',  ( -0.000000000000000000, 1.000000000000000000, -0.000000000000000000 ) ) ;
#4106=CARTESIAN_POINT ( 'NONE',  ( 37.16608720827707657, -51.86186943028246787, 57.49999999999999289 ) ) ;
#4126=VERTEX_POINT ( 'NONE', #25360 ) ;
#4136=DIRECTION ( 'NONE',  ( 0.000000000000000000, 0.000000000000000000, 1.000000000000000000 ) ) ;
#4140=CARTESIAN_POINT ( 'NONE',  ( -47.00000000000000000, 87.00000000000001421, 52.49999999999999289 ) ) ;
#4149=DIRECTION ( 'NONE',  ( 0.000000000000000000, 0.000000000000000000, 1.000000000000000000 ) ) ;
#4163=DIRECTION ( 'NONE',  ( 0.000000000000000000, 0.000000000000000000, -1.000000000000000000 ) ) ;
#4174=TOROIDAL_SURFACE ( 'NONE', #27614, 17.00000000000000000, 3.000000000000000000 ) ;
#4178=CIRCLE ( 'NONE', #7096, 7.500000000000013323 ) ;
#4198=FACE_OUTER_BOUND ( 'NONE', #20942, .T. ) ;
#4201=CARTESIAN_POINT ( 'NONE',  ( 39.99999999999998579, 0.000000000000000000, 62.49999999999999289 ) ) ;
#4202=DIRECTION ( 'NONE',  ( 1.000000000000000000, 0.000000000000000000, 0.000000000000000000 ) ) ;
#4216=VECTOR ( 'NONE', #30204, 1000.000000000000000 ) ;
#4225=ORIENTED_EDGE ( 'NONE', *, *, #9051, .T. ) ;
#4241=LINE ( 'NONE', #6445, #26813 ) ;
#4247=ADVANCED_FACE ( 'NONE', ( #528 ), #12297, .T. ) ;
#4260=EDGE_CURVE ( 'NONE', #4652, #6382, #12402, .T. ) ;
#4274=DIRECTION ( 'NONE',  ( 1.000000000000000000, 0.000000000000000000, 0.000000000000000000 ) ) ;
#4281=DIRECTION ( 'NONE',  ( 0.000000000000000000, 0.000000000000000000, -1.000000000000000000 ) ) ;
#4282=CARTESIAN_POINT ( 'NONE',  ( -41.18576677649696904, 67.96526564190969566, 12.55147014419179641 ) ) ;
#4285=FACE_OUTER_BOUND ( 'NONE', #13846, .T. ) ;
#4290=CARTESIAN_POINT ( 'NONE',  ( 49.99999999999998579, 90.00000000000001421, 62.49999999999999289 ) ) ;
#4318=VECTOR ( 'NONE', #22725, 1000.000000000000000 ) ;
#4321=FACE_OUTER_BOUND ( 'NONE', #25208, .T. ) ;
#4335=ORIENTED_EDGE ( 'NONE', *, *, #28125, .F. ) ;
#4336=CARTESIAN_POINT ( 'NONE',  ( -49.37764993206276642, 69.99068904741281472, 55.98768320531517872 ) ) ;
#4338=ORIENTED_EDGE ( 'NONE', *, *, #17404, .F. ) ;
#4343=CARTESIAN_POINT ( 'NONE',  ( 37.99999999999999289, 80.00000000000000000, 0.000000000000000000 ) ) ;
#4353=VECTOR ( 'NONE', #18024, 1000.000000000000000 ) ;
#4376=DIRECTION ( 'NONE',  ( -1.000000000000000000, 0.000000000000000000, -0.000000000000000000 ) ) ;
#4390=DIRECTION ( 'NONE',  ( -0.000000000000000000, 0.000000000000000000, -1.000000000000000000 ) ) ;
#4398=DIRECTION ( 'NONE',  ( -1.000000000000000000, 0.000000000000000000, 0.000000000000000000 ) ) ;
#4406=ADVANCED_FACE ( 'NONE', ( #15174 ), #8178, .T. ) ;
#4431=ADVANCED_FACE ( 'NONE', ( #1915 ), #9240, .T. ) ;
#4433=VECTOR ( 'NONE', #9673, 1000.000000000000000 ) ;
#4440=FACE_OUTER_BOUND ( 'NONE', #27615, .T. ) ;
#4445=DIRECTION ( 'NONE',  ( 0.000000000000000000, 0.000000000000000000, 1.000000000000000000 ) ) ;
#4447=CARTESIAN_POINT ( 'NONE',  ( 39.99999999999998579, 87.00000000000001421, 52.49999999999999289 ) ) ;
#4450=EDGE_LOOP ( 'NONE', ( #12033, #25018, #12184, #29434 ) ) ;
#4470=AXIS2_PLACEMENT_3D ( 'NONE', #28446, #18328, #30465 ) ;
#4483=ORIENTED_EDGE ( 'NONE', *, *, #3470, .F. ) ;
#4505=VERTEX_POINT ( 'NONE', #11134 ) ;
#4506=CIRCLE ( 'NONE', #25445, 7.500000000000000000 ) ;
#4513=VERTEX_POINT ( 'NONE', #4106 ) ;
#4521=AXIS2_PLACEMENT_3D ( 'NONE', #14643, #12939, #2794 ) ;
#4528=FACE_OUTER_BOUND ( 'NONE', #20639, .T. ) ;
#4532=CARTESIAN_POINT ( 'NONE',  ( 0.000000000000000000, 65.00000000000000000, 50.49999999999998579 ) ) ;
#4555=CARTESIAN_POINT ( 'NONE',  ( 42.49999999999998579, 50.00000000000000000, 12.49999999999999112 ) ) ;
#4566=FACE_OUTER_BOUND ( 'NONE', #26121, .T. ) ;
#4567=ORIENTED_EDGE ( 'NONE', *, *, #25632, .F. ) ;
#4572=CARTESIAN_POINT ( 'NONE',  ( 42.49999999999998579, -50.00000000000000000, 62.49999999999999289 ) ) ;
#4577=VERTEX_POINT ( 'NONE', #21863 ) ;
#4597=DIRECTION ( 'NONE',  ( -1.000000000000000000, 0.000000000000000000, 0.000000000000000000 ) ) ;
#4604=ORIENTED_EDGE ( 'NONE', *, *, #4988, .F. ) ;
#4606=FACE_OUTER_BOUND ( 'NONE', #1726, .T. ) ;
#4612=ORIENTED_EDGE ( 'NONE', *, *, #27152, .T. ) ;
#4640=ORIENTED_EDGE ( 'NONE', *, *, #7718, .T. ) ;
#4646=EDGE_CURVE ( 'NONE', #2167, #12762, #23762, .T. ) ;
#4647=ORIENTED_EDGE ( 'NONE', *, *, #26147, .T. ) ;
#4652=VERTEX_POINT ( 'NONE', #14061 ) ;
#4658=ORIENTED_EDGE ( 'NONE', *, *, #21962, .F. ) ;
#4662=EDGE_CURVE ( 'NONE', #15798, #20585, #18798, .T. ) ;
#4664=LINE ( 'NONE', #3243, #11611 ) ;
#4689=DIRECTION ( 'NONE',  ( 0.000000000000000000, 0.000000000000000000, -1.000000000000000000 ) ) ;
#4710=CARTESIAN_POINT ( 'NONE',  ( -2.081668171172168513E-14, 80.00000000000000000, 37.49999999999999289 ) ) ;
#4719=CARTESIAN_POINT ( 'NONE',  ( 37.16608720827707657, -65.00000000000000000, 97.07879600563551037 ) ) ;
#4731=ORIENTED_EDGE ( 'NONE', *, *, #8208, .F. ) ;
#4738=DIRECTION ( 'NONE',  ( -0.000000000000000000, -0.000000000000000000, 1.000000000000000000 ) ) ;
#4748=EDGE_CURVE ( 'NONE', #19059, #20079, #13400, .T. ) ;
#4763=DIRECTION ( 'NONE',  ( 0.000000000000000000, 0.000000000000000000, -1.000000000000000000 ) ) ;
#4765=ORIENTED_EDGE ( 'NONE', *, *, #23833, .T. ) ;
#4776=CARTESIAN_POINT ( 'NONE',  ( -64.99999999999998579, 36.86186943028246787, 12.49999999999999112 ) ) ;
#4780=CYLINDRICAL_SURFACE ( 'NONE', #7047, 3.000000000000002665 ) ;
#4783=ORIENTED_EDGE ( 'NONE', *, *, #20862, .T. ) ;
#4788=ORIENTED_EDGE ( 'NONE', *, *, #6550, .T. ) ;
#4811=VECTOR ( 'NONE', #14610, 1000.000000000000000 ) ;
#4813=FACE_OUTER_BOUND ( 'NONE', #2331, .T. ) ;
#4817=CARTESIAN_POINT ( 'NONE',  ( -40.00000000000002842, 80.00000000000001421, 27.49999999999983658 ) ) ;
#4822=DIRECTION ( 'NONE',  ( -0.000000000000000000, -0.000000000000000000, 1.000000000000000000 ) ) ;
#4849=CIRCLE ( 'NONE', #26266, 5.000000000000004441 ) ;
#4862=VERTEX_POINT ( 'NONE', #21824 ) ;
#4923=CIRCLE ( 'NONE', #9886, 50.00000000000000000 ) ;
#4925=EDGE_LOOP ( 'NONE', ( #28982, #987, #26981, #872 ) ) ;
#4928=EDGE_CURVE ( 'NONE', #25203, #10854, #5137, .T. ) ;
#4951=VECTOR ( 'NONE', #10605, 1000.000000000000000 ) ;
#4962=ORIENTED_EDGE ( 'NONE', *, *, #30551, .F. ) ;
#4980=VERTEX_POINT ( 'NONE', #28856 ) ;
#4988=EDGE_CURVE ( 'NONE', #21772, #15921, #19174, .T. ) ;
#4999=DIRECTION ( 'NONE',  ( -1.000000000000000000, 0.000000000000000000, 0.000000000000000000 ) ) ;
#5004=ORIENTED_EDGE ( 'NONE', *, *, #3097, .T. ) ;
#5005=ADVANCED_FACE ( 'NONE', ( #5101 ), #28810, .T. ) ;
#5009=VERTEX_POINT ( 'NONE', #27085 ) ;
#5013=DIRECTION ( 'NONE',  ( 0.000000000000000000, 0.000000000000000000, -1.000000000000000000 ) ) ;
#5029=DIRECTION ( 'NONE',  ( -0.000000000000000000, 1.000000000000000000, -0.000000000000000000 ) ) ;
#5037=ORIENTED_EDGE ( 'NONE', *, *, #20349, .F. ) ;
#5048=EDGE_LOOP ( 'NONE', ( #9836, #284, #24707, #405, #25214 ) ) ;
#5053=CARTESIAN_POINT ( 'NONE',  ( 0.000000000000000000, 0.000000000000000000, 92.49999999999998579 ) ) ;
#5069=DIRECTION ( 'NONE',  ( -0.000000000000000000, 1.000000000000000000, -0.000000000000000000 ) ) ;
#5070=CARTESIAN_POINT ( 'NONE',  ( 37.16608720827707657, 51.86186943028246787, 97.07879600563551037 ) ) ;
#5073=CARTESIAN_POINT ( 'NONE',  ( -40.00000000000000000, 90.00000000000001421, 59.49999999999999289 ) ) ;
#5076=VECTOR ( 'NONE', #21496, 1000.000000000000000 ) ;
#5078=VERTEX_POINT ( 'NONE', #17102 ) ;
#5093=ORIENTED_EDGE ( 'NONE', *, *, #10026, .F. ) ;
#5101=FACE_OUTER_BOUND ( 'NONE', #8027, .T. ) ;
#5102=LINE ( 'NONE', #14613, #3038 ) ;
#5104=ORIENTED_EDGE ( 'NONE', *, *, #17397, .F. ) ;
#5105=FACE_OUTER_BOUND ( 'NONE', #4450, .T. ) ;
#5109=DIRECTION ( 'NONE',  ( 0.000000000000000000, 0.000000000000000000, 1.000000000000000000 ) ) ;
#5137=LINE ( 'NONE', #2493, #21771 ) ;
#5139=VERTEX_POINT ( 'NONE', #3376 ) ;
#5147=VECTOR ( 'NONE', #26430, 1000.000000000000000 ) ;
#5157=UNCERTAINTY_MEASURE_WITH_UNIT (LENGTH_MEASURE( 1.000000000000000082E-05 ), #433, 'distance_accuracy_value', 'NONE');
#5166=DIRECTION ( 'NONE',  ( 0.000000000000000000, -0.000000000000000000, -1.000000000000000000 ) ) ;
#5173=DIRECTION ( 'NONE',  ( 0.000000000000000000, 0.000000000000000000, 1.000000000000000000 ) ) ;
#5174=CARTESIAN_POINT ( 'NONE',  ( 34.99999999999933920, 4.286263797015655244E-15, 92.49999999999998579 ) ) ;
#5181=ADVANCED_FACE ( 'NONE', ( #22691, #22856 ), #15842, .T. ) ;
#5187=ADVANCED_FACE ( 'NONE', ( #8374 ), #27235, .T. ) ;
#5206=EDGE_CURVE ( 'NONE', #3904, #26649, #2876, .T. ) ;
#5212=DIRECTION ( 'NONE',  ( 0.000000000000000000, 0.000000000000000000, 1.000000000000000000 ) ) ;
#5215=ORIENTED_EDGE ( 'NONE', *, *, #21350, .F. ) ;
#5222=EDGE_CURVE ( 'NONE', #23472, #5078, #9844, .T. ) ;
#5224=DIRECTION ( 'NONE',  ( -1.000000000000000000, 0.000000000000000000, 0.000000000000000000 ) ) ;
#5242=FACE_OUTER_BOUND ( 'NONE', #28065, .T. ) ;
#5252=DIRECTION ( 'NONE',  ( 1.000000000000000000, 0.000000000000000000, 0.000000000000000000 ) ) ;
#5275=EDGE_LOOP ( 'NONE', ( #19433, #28369, #19966, #29124 ) ) ;
#5286=CYLINDRICAL_SURFACE ( 'NONE', #4521, 45.00000000000000711 ) ;
#5287=CARTESIAN_POINT ( 'NONE',  ( 69.99999999999998579, -50.00000000000000000, 59.49999999999999289 ) ) ;
#5291=AXIS2_PLACEMENT_3D ( 'NONE', #23203, #1857, #18695 ) ;
#5327=DIRECTION ( 'NONE',  ( 0.000000000000000000, 0.000000000000000000, -1.000000000000000000 ) ) ;
#5343=ORIENTED_EDGE ( 'NONE', *, *, #30546, .F. ) ;
#5356=EDGE_LOOP ( 'NONE', ( #7772, #14650, #7406, #29746 ) ) ;
#5359=CARTESIAN_POINT ( 'NONE',  ( 4.510281037539698445E-13, -4.926614671774132148E-13, 79.49999999999998579 ) ) ;
#5393=ORIENTED_EDGE ( 'NONE', *, *, #18135, .T. ) ;
#5395=ADVANCED_FACE ( 'NONE', ( #4285 ), #9590, .F. ) ;
#5397=CARTESIAN_POINT ( 'NONE',  ( -40.00000000000002842, 80.00000000000001421, 52.50000000000014921 ) ) ;
#5422=ORIENTED_EDGE ( 'NONE', *, *, #25429, .F. ) ;
#5435=VECTOR ( 'NONE', #14219, 1000.000000000000000 ) ;
#5436=CYLINDRICAL_SURFACE ( 'NONE', #27723, 3.000000000000002665 ) ;
#5440=ORIENTED_EDGE ( 'NONE', *, *, #26578, .F. ) ;
#5464=DIRECTION ( 'NONE',  ( 1.000000000000000000, 0.000000000000000000, 0.000000000000000000 ) ) ;
#5466=VERTEX_POINT ( 'NONE', #24392 ) ;
#5469=CARTESIAN_POINT ( 'NONE',  ( 37.16608720827707657, -36.86186943028246787, 57.49999999999999289 ) ) ;
#5476=AXIS2_PLACEMENT_3D ( 'NONE', #1515, #5719, #1356 ) ;
#5530=CARTESIAN_POINT ( 'NONE',  ( -57.50000000000001421, -50.00000000000000000, 97.07879600563551037 ) ) ;
#5539=DIRECTION ( 'NONE',  ( 1.000000000000000000, 0.000000000000000000, 0.000000000000000000 ) ) ;
#5540=EDGE_CURVE ( 'NONE', #4862, #26649, #11573, .T. ) ;
#5541=ORIENTED_EDGE ( 'NONE', *, *, #1572, .T. ) ;
#5551=FACE_BOUND ( 'NONE', #6686, .T. ) ;
#5552=CARTESIAN_POINT ( 'NONE',  ( 39.99999999999998579, 80.00000000000001421, 17.49999999999999645 ) ) ;
#5556=ADVANCED_FACE ( 'NONE', ( #3338 ), #20487, .T. ) ;
#5559=DIRECTION ( 'NONE',  ( 0.000000000000000000, -1.000000000000000000, 0.000000000000000000 ) ) ;
#5563=CARTESIAN_POINT ( 'NONE',  ( -42.49999999999998579, -50.00000000000000000, 62.49999999999999289 ) ) ;
#5601=AXIS2_PLACEMENT_3D ( 'NONE', #13314, #4097, #3958 ) ;
#5612=ORIENTED_EDGE ( 'NONE', *, *, #865, .T. ) ;
#5620=ORIENTED_EDGE ( 'NONE', *, *, #10768, .T. ) ;
#5628=ORIENTED_EDGE ( 'NONE', *, *, #27520, .F. ) ;
#5630=ORIENTED_EDGE ( 'NONE', *, *, #17536, .T. ) ;
#5665=DIRECTION ( 'NONE',  ( -1.000000000000000000, 0.000000000000000000, 0.000000000000000000 ) ) ;
#5701=CARTESIAN_POINT ( 'NONE',  ( -38.00000000000000000, 65.00000000000000000, 15.49999999999998579 ) ) ;
#5711=CIRCLE ( 'NONE', #14674, 5.000000000000004441 ) ;
#5715=LINE ( 'NONE', #15208, #8306 ) ;
#5719=DIRECTION ( 'NONE',  ( 0.000000000000000000, 0.000000000000000000, -1.000000000000000000 ) ) ;
#5744=CARTESIAN_POINT ( 'NONE',  ( 42.49999999999998579, -50.00000000000000000, 97.07879600563551037 ) ) ;
#5751=VERTEX_POINT ( 'NONE', #13096 ) ;
#5774=CARTESIAN_POINT ( 'NONE',  ( 14.99999999999995737, 1.387778780781445676E-14, 92.49999999999998579 ) ) ;
#5784=DIRECTION ( 'NONE',  ( 0.000000000000000000, 1.000000000000000000, 0.000000000000000000 ) ) ;
#5791=VERTEX_POINT ( 'NONE', #10441 ) ;
#5801=EDGE_CURVE ( 'NONE', #5466, #21772, #19060, .T. ) ;
#5803=DIRECTION ( 'NONE',  ( -1.000000000000000000, 0.000000000000000000, 0.000000000000000000 ) ) ;
#5829=LINE ( 'NONE', #833, #8130 ) ;
#5834=AXIS2_PLACEMENT_3D ( 'NONE', #21080, #25487, #25637 ) ;
#5841=DIRECTION ( 'NONE',  ( -0.000000000000000000, 1.000000000000000000, -0.000000000000000000 ) ) ;
#5854=CIRCLE ( 'NONE', #6345, 3.000000000000002665 ) ;
#5861=DIRECTION ( 'NONE',  ( 0.000000000000000000, -1.000000000000000000, 0.000000000000000000 ) ) ;
#5875=CYLINDRICAL_SURFACE ( 'NONE', #1841, 2.999999999999999112 ) ;
#5876=DIRECTION ( 'NONE',  ( 1.000000000000000000, 0.000000000000000000, 0.000000000000000000 ) ) ;
#5880=CIRCLE ( 'NONE', #14820, 20.00000000000000355 ) ;
#5887=CARTESIAN_POINT ( 'NONE',  ( 37.16608720827707657, -65.00000000000000000, 12.49999999999999112 ) ) ;
#5888=ORIENTED_EDGE ( 'NONE', *, *, #2882, .F. ) ;
#5899=DIRECTION ( 'NONE',  ( -0.000000000000000000, 0.000000000000000000, 1.000000000000000000 ) ) ;
#5911=EDGE_LOOP ( 'NONE', ( #921, #16729, #4788, #17379 ) ) ;
#5944=LINE ( 'NONE', #8457, #20790 ) ;
#5955=VECTOR ( 'NONE', #22061, 1000.000000000000000 ) ;
#5956=CARTESIAN_POINT ( 'NONE',  ( 42.15079010498045875, 66.40049817264792864, 62.28254144336177944 ) ) ;
#5980=DIRECTION ( 'NONE',  ( 0.000000000000000000, 0.000000000000000000, -1.000000000000000000 ) ) ;
#5998=CYLINDRICAL_SURFACE ( 'NONE', #15904, 15.00000000000000000 ) ;
#6007=DIRECTION ( 'NONE',  ( -1.000000000000000000, 0.000000000000000000, 0.000000000000000000 ) ) ;
#6015=DIRECTION ( 'NONE',  ( 0.000000000000000000, 0.000000000000000000, 1.000000000000000000 ) ) ;
#6016=EDGE_LOOP ( 'NONE', ( #7658, #1225, #30802, #28376, #8126, #10649, #14585, #14876 ) ) ;
#6032=CARTESIAN_POINT ( 'NONE',  ( 0.000000000000000000, 0.000000000000000000, 12.49999999999999112 ) ) ;
#6043=DIRECTION ( 'NONE',  ( 0.000000000000000000, 0.000000000000000000, -1.000000000000000000 ) ) ;
#6054=LINE ( 'NONE', #25080, #29279 ) ;
#6055=LINE ( 'NONE', #15564, #5147 ) ;
#6061=CYLINDRICAL_SURFACE ( 'NONE', #6822, 7.500000000000000000 ) ;
#6067=CARTESIAN_POINT ( 'NONE',  ( 42.08856419149575601, 68.37167730218320116, 12.71573695841679985 ) ) ;
#6068=CYLINDRICAL_SURFACE ( 'NONE', #30052, 45.00000000000000711 ) ;
#6073=DIRECTION ( 'NONE',  ( 1.000000000000000000, 0.000000000000000000, -0.000000000000000000 ) ) ;
#6085=EDGE_CURVE ( 'NONE', #18, #12762, #11814, .T. ) ;
#6090=ORIENTED_EDGE ( 'NONE', *, *, #7080, .F. ) ;
#6095=CARTESIAN_POINT ( 'NONE',  ( 39.99999999999998579, 80.00000000000001421, 57.49999999999998579 ) ) ;
#6115=EDGE_CURVE ( 'NONE', #15627, #15944, #23026, .T. ) ;
#6141=AXIS2_PLACEMENT_3D ( 'NONE', #25826, #28624, #11626 ) ;
#6145=ORIENTED_EDGE ( 'NONE', *, *, #22910, .T. ) ;
#6159=VECTOR ( 'NONE', #28989, 1000.000000000000000 ) ;
#6165=CIRCLE ( 'NONE', #29567, 45.00000000000000711 ) ;
#6187=AXIS2_PLACEMENT_3D ( 'NONE', #20381, #4149, #3849 ) ;
#6189=EDGE_CURVE ( 'NONE', #1222, #2571, #22406, .T. ) ;
#6190=CARTESIAN_POINT ( 'NONE',  ( 49.99999999999998579, -50.00000000000000000, 59.49999999999999289 ) ) ;
#6191=ORIENTED_EDGE ( 'NONE', *, *, #2901, .T. ) ;
#6196=ORIENTED_EDGE ( 'NONE', *, *, #19905, .F. ) ;
#6217=ORIENTED_EDGE ( 'NONE', *, *, #17597, .T. ) ;
#6221=VERTEX_POINT ( 'NONE', #21939 ) ;
#6229=VECTOR ( 'NONE', #17548, 1000.000000000000000 ) ;
#6232=DIRECTION ( 'NONE',  ( 0.000000000000000000, 0.000000000000000000, -1.000000000000000000 ) ) ;
#6257=FACE_OUTER_BOUND ( 'NONE', #26474, .T. ) ;
#6264=CARTESIAN_POINT ( 'NONE',  ( -50.00000000000000000, 70.00000000000000000, 12.49999999999999112 ) ) ;
#6271=ORIENTED_EDGE ( 'NONE', *, *, #13466, .F. ) ;
#6277=DIRECTION ( 'NONE',  ( 0.000000000000000000, -0.000000000000000000, -1.000000000000000000 ) ) ;
#6280=FACE_OUTER_BOUND ( 'NONE', #10225, .T. ) ;
#6288=CARTESIAN_POINT ( 'NONE',  ( 52.16608720827707657, 51.86186943028246787, 97.07879600563551037 ) ) ;
#6324=CARTESIAN_POINT ( 'NONE',  ( 46.99999999999998579, 90.00000000000001421, 52.49999999999999289 ) ) ;
#6329=ADVANCED_FACE ( 'NONE', ( #23005 ), #11173, .F. ) ;
#6345=AXIS2_PLACEMENT_3D ( 'NONE', #10278, #21979, #19957 ) ;
#6347=DIRECTION ( 'NONE',  ( -1.000000000000000000, 0.000000000000000000, 0.000000000000000000 ) ) ;
#6350=ORIENTED_EDGE ( 'NONE', *, *, #13012, .F. ) ;
#6360=AXIS2_PLACEMENT_3D ( 'NONE', #14982, #21851, #5166 ) ;
#6382=VERTEX_POINT ( 'NONE', #14251 ) ;
#6384=CARTESIAN_POINT ( 'NONE',  ( 39.99999999999998579, 67.32050807568877815, 12.49999999999999112 ) ) ;
#6386=CARTESIAN_POINT ( 'NONE',  ( 0.000000000000000000, 0.000000000000000000, 82.49999999999998579 ) ) ;
#6404=DIRECTION ( 'NONE',  ( 0.000000000000000000, 0.000000000000000000, -1.000000000000000000 ) ) ;
#6407=ORIENTED_EDGE ( 'NONE', *, *, #6693, .T. ) ;
#6408=AXIS2_PLACEMENT_3D ( 'NONE', #8166, #15477, #5665 ) ;
#6445=CARTESIAN_POINT ( 'NONE',  ( -37.16608720827707657, 65.00000000000000000, 97.07879600563551037 ) ) ;
#6448=EDGE_CURVE ( 'NONE', #9580, #15627, #24524, .T. ) ;
#6479=ORIENTED_EDGE ( 'NONE', *, *, #395, .F. ) ;
#6486=CARTESIAN_POINT ( 'NONE',  ( -4.163336342344337027E-14, 1.387778780781445676E-14, 67.49999999999997158 ) ) ;
#6495=CARTESIAN_POINT ( 'NONE',  ( -50.00000000000000000, 50.00000000000000000, 59.49999999999999289 ) ) ;
#6505=ADVANCED_FACE ( 'NONE', ( #19106 ), #30800, .T. ) ;
#6518=ADVANCED_FACE ( 'NONE', ( #23321 ), #28325, .F. ) ;
#6519=DIRECTION ( 'NONE',  ( 0.000000000000000000, 0.000000000000000000, 1.000000000000000000 ) ) ;
#6530=EDGE_CURVE ( 'NONE', #7224, #20725, #10204, .T. ) ;
#6535=VECTOR ( 'NONE', #15957, 1000.000000000000000 ) ;
#6550=EDGE_CURVE ( 'NONE', #10235, #19317, #10055, .T. ) ;
#6569=CIRCLE ( 'NONE', #20501, 45.00000000000000711 ) ;
#6576=EDGE_CURVE ( 'NONE', #18, #8092, #7632, .T. ) ;
#6584=DIRECTION ( 'NONE',  ( 0.000000000000000000, 0.000000000000000000, -1.000000000000000000 ) ) ;
#6589=CARTESIAN_POINT ( 'NONE',  ( 49.99999999999998579, 50.00000000000000000, 62.49999999999999289 ) ) ;
#6590=CARTESIAN_POINT ( 'NONE',  ( 49.99999999999999289, 70.00000000000001421, 53.15267136187731722 ) ) ;
#6598=DIRECTION ( 'NONE',  ( -1.000000000000000000, 0.000000000000000000, 0.000000000000000000 ) ) ;
#6605=ORIENTED_EDGE ( 'NONE', *, *, #9706, .T. ) ;
#6622=ORIENTED_EDGE ( 'NONE', *, *, #11194, .F. ) ;
#6624=CARTESIAN_POINT ( 'NONE',  ( 35.41742430504415040, 80.00000000000000000, 50.49999999999998579 ) ) ;
#6630=VECTOR ( 'NONE', #14583, 1000.000000000000000 ) ;
#6648=VECTOR ( 'NONE', #13893, 1000.000000000000000 ) ;
#6654=ORIENTED_EDGE ( 'NONE', *, *, #15509, .F. ) ;
#6661=CYLINDRICAL_SURFACE ( 'NONE', #19066, 15.00000000000000000 ) ;
#6670=AXIS2_PLACEMENT_3D ( 'NONE', #3141, #27928, #6404 ) ;
#6673=ORIENTED_EDGE ( 'NONE', *, *, #18952, .T. ) ;
#6678=DIRECTION ( 'NONE',  ( -1.000000000000000000, 0.000000000000000000, 0.000000000000000000 ) ) ;
#6679=ORIENTED_EDGE ( 'NONE', *, *, #14496, .T. ) ;
#6686=EDGE_LOOP ( 'NONE', ( #4658, #30851 ) ) ;
#6693=EDGE_CURVE ( 'NONE', #4980, #10762, #23554, .T. ) ;
#6697=DIRECTION ( 'NONE',  ( 0.000000000000000000, 0.000000000000000000, 1.000000000000000000 ) ) ;
#6707=VECTOR ( 'NONE', #22221, 1000.000000000000000 ) ;
#6708=PLANE ( 'NONE',  #8841 ) ;
#6726=DIRECTION ( 'NONE',  ( -1.000000000000000000, 0.000000000000000000, 0.000000000000000000 ) ) ;
#6733=AXIS2_PLACEMENT_3D ( 'NONE', #22142, #17000, #4999 ) ;
#6735=CARTESIAN_POINT ( 'NONE',  ( -50.00000000000000000, 87.00000000000001421, 52.49999999999999289 ) ) ;
#6742=EDGE_CURVE ( 'NONE', #14629, #11642, #22509, .T. ) ;
#6743=EDGE_CURVE ( 'NONE', #5791, #19317, #23045, .T. ) ;
#6754=CIRCLE ( 'NONE', #1796, 50.00000000000000000 ) ;
#6763=CIRCLE ( 'NONE', #10257, 15.00000000000000000 ) ;
#6764=DIRECTION ( 'NONE',  ( 0.000000000000000000, -1.000000000000000000, 0.000000000000000000 ) ) ;
#6773=DIRECTION ( 'NONE',  ( 0.000000000000000000, 0.000000000000000000, -1.000000000000000000 ) ) ;
#6810=CARTESIAN_POINT ( 'NONE',  ( -4.163336342344337027E-14, 1.387778780781445676E-14, 77.49999999999998579 ) ) ;
#6814=DIRECTION ( 'NONE',  ( 0.000000000000000000, -1.000000000000000000, 0.000000000000000000 ) ) ;
#6816=DIRECTION ( 'NONE',  ( 0.000000000000000000, 0.000000000000000000, -1.000000000000000000 ) ) ;
#6822=AXIS2_PLACEMENT_3D ( 'NONE', #24935, #13816, #4597 ) ;
#6833=ORIENTED_EDGE ( 'NONE', *, *, #28102, .F. ) ;
#6834=FACE_OUTER_BOUND ( 'NONE', #23666, .T. ) ;
#6838=AXIS2_PLACEMENT_3D ( 'NONE', #10223, #15361, #869 ) ;
#6840=FACE_OUTER_BOUND ( 'NONE', #18554, .T. ) ;
#6862=AXIS2_PLACEMENT_3D ( 'NONE', #13803, #16444, #11467 ) ;
#6879=CARTESIAN_POINT ( 'NONE',  ( 29.99999999999925038, 1.387778780781445676E-14, 67.49999999999997158 ) ) ;
#6897=ADVANCED_FACE ( 'NONE', ( #4566 ), #30309, .T. ) ;
#6898=DIRECTION ( 'NONE',  ( -1.000000000000000000, 0.000000000000000000, 0.000000000000000000 ) ) ;
#6912=CIRCLE ( 'NONE', #3442, 3.000000000000002665 ) ;
#6916=DIRECTION ( 'NONE',  ( 1.000000000000000000, 0.000000000000000000, 0.000000000000000000 ) ) ;
#6924=ORIENTED_EDGE ( 'NONE', *, *, #16803, .F. ) ;
#6926=FACE_OUTER_BOUND ( 'NONE', #24397, .T. ) ;
#6941=DIRECTION ( 'NONE',  ( 0.000000000000000000, 0.000000000000000000, -1.000000000000000000 ) ) ;
#6968=DIRECTION ( 'NONE',  ( -1.000000000000000000, 0.000000000000000000, 0.000000000000000000 ) ) ;
#6976=LINE ( 'NONE', #19440, #9864 ) ;
#6997=AXIS2_PLACEMENT_3D ( 'NONE', #14940, #20229, #29136 ) ;
#6999=DIRECTION ( 'NONE',  ( -0.000000000000000000, -0.000000000000000000, 1.000000000000000000 ) ) ;
#7000=ADVANCED_FACE ( 'NONE', ( #12985 ), #22476, .T. ) ;
#7004=EDGE_LOOP ( 'NONE', ( #12119, #28440, #2198, #26956, #22573 ) ) ;
#7006=DIRECTION ( 'NONE',  ( -0.000000000000000000, 1.000000000000000000, -0.000000000000000000 ) ) ;
#7022=CARTESIAN_POINT ( 'NONE',  ( 39.99999999999998579, 90.00000000000001421, 17.49999999999999645 ) ) ;
#7040=LINE ( 'NONE', #28566, #2313 ) ;
#7044=CARTESIAN_POINT ( 'NONE',  ( -37.16608720827707657, -51.86186943028246787, 57.49999999999999289 ) ) ;
#7047=AXIS2_PLACEMENT_3D ( 'NONE', #21147, #6816, #11656 ) ;
#7052=ORIENTED_EDGE ( 'NONE', *, *, #16994, .T. ) ;
#7061=CARTESIAN_POINT ( 'NONE',  ( 46.99999999999998579, 87.00000000000001421, 52.49999999999999289 ) ) ;
#7073=ORIENTED_EDGE ( 'NONE', *, *, #15862, .T. ) ;
#7078=ORIENTED_EDGE ( 'NONE', *, *, #17433, .T. ) ;
#7080=EDGE_CURVE ( 'NONE', #10893, #19850, #29568, .T. ) ;
#7095=DIRECTION ( 'NONE',  ( -1.000000000000000000, 0.000000000000000000, 0.000000000000000000 ) ) ;
#7096=AXIS2_PLACEMENT_3D ( 'NONE', #14892, #24401, #3045 ) ;
#7108=EDGE_CURVE ( 'NONE', #5078, #23472, #13643, .T. ) ;
#7109=CARTESIAN_POINT ( 'NONE',  ( -50.00000000000000000, 87.00000000000001421, 22.49999999999999289 ) ) ;
#7135=CARTESIAN_POINT ( 'NONE',  ( 66.99999999999998579, -50.00000000000000000, 59.49999999999999289 ) ) ;
#7148=DIRECTION ( 'NONE',  ( 0.000000000000000000, 0.000000000000000000, -1.000000000000000000 ) ) ;
#7152=ORIENTED_EDGE ( 'NONE', *, *, #9031, .T. ) ;
#7179=DIRECTION ( 'NONE',  ( 0.000000000000000000, -1.000000000000000000, 0.000000000000000000 ) ) ;
#7193=ORIENTED_EDGE ( 'NONE', *, *, #20037, .F. ) ;
#7199=CARTESIAN_POINT ( 'NONE',  ( 4.510281037539698445E-13, -4.926614671774132148E-13, 79.49999999999998579 ) ) ;
#7200=CARTESIAN_POINT ( 'NONE',  ( 4.510281037539698445E-13, -4.926614671774132148E-13, 62.49999999999999289 ) ) ;
#7205=ORIENTED_EDGE ( 'NONE', *, *, #27671, .T. ) ;
#7224=VERTEX_POINT ( 'NONE', #3 ) ;
#7230=ORIENTED_EDGE ( 'NONE', *, *, #4646, .F. ) ;
#7235=FACE_OUTER_BOUND ( 'NONE', #5911, .T. ) ;
#7243=CARTESIAN_POINT ( 'NONE',  ( -37.16608720827707657, 65.00000000000000000, 57.49999999999999289 ) ) ;
#7249=ORIENTED_EDGE ( 'NONE', *, *, #12056, .T. ) ;
#7294=CARTESIAN_POINT ( 'NONE',  ( -49.67292458505995256, 69.99754304297013618, 55.05739345352110803 ) ) ;
#7299=FACE_OUTER_BOUND ( 'NONE', #10670, .T. ) ;
#7301=AXIS2_PLACEMENT_3D ( 'NONE', #4343, #9039, #6232 ) ;
#7307=VECTOR ( 'NONE', #17064, 1000.000000000000000 ) ;
#7317=AXIS2_PLACEMENT_3D ( 'NONE', #19749, #9941, #21938 ) ;
#7335=ORIENTED_EDGE ( 'NONE', *, *, #19531, .F. ) ;
#7343=CIRCLE ( 'NONE', #24760, 7.500000000000000000 ) ;
#7346=CIRCLE ( 'NONE', #11341, 3.000000000000002665 ) ;
#7367=CARTESIAN_POINT ( 'NONE',  ( 34.99999999999933920, 4.286263797015655244E-15, 85.49999999999998579 ) ) ;
#7385=DIRECTION ( 'NONE',  ( 0.000000000000000000, 1.000000000000000000, 0.000000000000000000 ) ) ;
#7386=ORIENTED_EDGE ( 'NONE', *, *, #10728, .F. ) ;
#7391=VERTEX_POINT ( 'NONE', #15733 ) ;
#7396=AXIS2_PLACEMENT_3D ( 'NONE', #9486, #28514, #21014 ) ;
#7401=ORIENTED_EDGE ( 'NONE', *, *, #13724, .T. ) ;
#7405=DIRECTION ( 'NONE',  ( -1.000000000000000000, 0.000000000000000000, 0.000000000000000000 ) ) ;
#7406=ORIENTED_EDGE ( 'NONE', *, *, #11303, .F. ) ;
#7425=VECTOR ( 'NONE', #23088, 1000.000000000000000 ) ;
#7426=DIRECTION ( 'NONE',  ( 0.000000000000000000, 0.000000000000000000, -1.000000000000000000 ) ) ;
#7436=ADVANCED_FACE ( 'NONE', ( #29481 ), #20104, .F. ) ;
#7446=EDGE_CURVE ( 'NONE', #17807, #21378, #3899, .T. ) ;
#7447=DIRECTION ( 'NONE',  ( -1.000000000000000000, 0.000000000000000000, 0.000000000000000000 ) ) ;
#7454=CARTESIAN_POINT ( 'NONE',  ( -50.00000000000000000, -50.00000000000000000, 62.49999999999999289 ) ) ;
#7459=ORIENTED_EDGE ( 'NONE', *, *, #24027, .T. ) ;
#7464=CARTESIAN_POINT ( 'NONE',  ( -65.00000000000000000, -36.86186943028246787, 57.49999999999999289 ) ) ;
#7465=VERTEX_POINT ( 'NONE', #13424 ) ;
#7475=ORIENTED_EDGE ( 'NONE', *, *, #24487, .F. ) ;
#7480=EDGE_CURVE ( 'NONE', #9580, #12801, #932, .T. ) ;
#7518=DIRECTION ( 'NONE',  ( 0.000000000000000000, 0.000000000000000000, 1.000000000000000000 ) ) ;
#7525=LINE ( 'NONE', #5174, #17247 ) ;
#7528=ORIENTED_EDGE ( 'NONE', *, *, #14712, .F. ) ;
#7556=DIRECTION ( 'NONE',  ( -0.000000000000000000, -0.000000000000000000, 1.000000000000000000 ) ) ;
#7558=CARTESIAN_POINT ( 'NONE',  ( -1.897971151300065476E-14, 90.00000000000001421, 22.49999999999999289 ) ) ;
#7559=EDGE_LOOP ( 'NONE', ( #26576, #13695, #24618, #2013 ) ) ;
#7561=DIRECTION ( 'NONE',  ( 0.000000000000000000, 0.000000000000000000, 1.000000000000000000 ) ) ;
#7573=DIRECTION ( 'NONE',  ( -1.000000000000000000, 0.000000000000000000, 0.000000000000000000 ) ) ;
#7578=PRODUCT_CONTEXT ( 'NONE', #3601, 'mechanical' ) ;
#7605=LINE ( 'NONE', #17432, #14636 ) ;
#7606=DIRECTION ( 'NONE',  ( 0.000000000000000000, 1.000000000000000000, 0.000000000000000000 ) ) ;
#7632=CIRCLE ( 'NONE', #3653, 7.500000000000000000 ) ;
#7646=EDGE_CURVE ( 'NONE', #26649, #24670, #21285, .T. ) ;
#7657=CIRCLE ( 'NONE', #15619, 15.00000000000000000 ) ;
#7658=ORIENTED_EDGE ( 'NONE', *, *, #25429, .T. ) ;
#7664=CARTESIAN_POINT ( 'NONE',  ( 48.00277007997793532, 69.90319682561420223, 58.53084797575039744 ) ) ;
#7672=ORIENTED_EDGE ( 'NONE', *, *, #11194, .T. ) ;
#7676=CARTESIAN_POINT ( 'NONE',  ( 39.99999999999998579, 90.00000000000001421, 52.49999999999999289 ) ) ;
#7683=CARTESIAN_POINT ( 'NONE',  ( -45.56537993551197019, 69.19660983124860820, 60.81053982466166730 ) ) ;
#7703=ORIENTED_EDGE ( 'NONE', *, *, #13800, .F. ) ;
#7718=EDGE_CURVE ( 'NONE', #7224, #16079, #21751, .T. ) ;
#7736=PLANE ( 'NONE',  #19161 ) ;
#7749=VECTOR ( 'NONE', #3127, 1000.000000000000000 ) ;
#7750=FACE_OUTER_BOUND ( 'NONE', #3071, .T. ) ;
#7756=EDGE_LOOP ( 'NONE', ( #22981, #27321, #12995, #20912 ) ) ;
#7772=ORIENTED_EDGE ( 'NONE', *, *, #23123, .F. ) ;
#7780=CIRCLE ( 'NONE', #23213, 4.999999999999997335 ) ;
#7788=ORIENTED_EDGE ( 'NONE', *, *, #27181, .T. ) ;
#7801=EDGE_CURVE ( 'NONE', #22741, #17807, #4178, .T. ) ;
#7829=VECTOR ( 'NONE', #8528, 1000.000000000000000 ) ;
#7832=CARTESIAN_POINT ( 'NONE',  ( -42.15079822434952916, 66.40050670621626239, 62.28253961994978738 ) ) ;
#7854=CIRCLE ( 'NONE', #8354, 15.00000000000000000 ) ;
#7862=VERTEX_POINT ( 'NONE', #13649 ) ;
#7863=EDGE_CURVE ( 'NONE', #2852, #11596, #11147, .T. ) ;
#7898=FACE_OUTER_BOUND ( 'NONE', #18543, .T. ) ;
#7934=ORIENTED_EDGE ( 'NONE', *, *, #27856, .F. ) ;
#7940=EDGE_LOOP ( 'NONE', ( #18521, #8804 ) ) ;
#7956=FACE_OUTER_BOUND ( 'NONE', #14159, .T. ) ;
#7963=PRODUCT ( 'Housing  Cover Cap', 'Housing  Cover Cap', '', ( #7578 ) ) ;
#7976=ORIENTED_EDGE ( 'NONE', *, *, #19143, .F. ) ;
#7985=CARTESIAN_POINT ( 'NONE',  ( 47.59023918323793367, 69.85947342368727675, 59.04212144534069040 ) ) ;
#7996=CARTESIAN_POINT ( 'NONE',  ( 43.96625041971210379, 68.08819673771459691, 61.68659123583229587 ) ) ;
#8027=EDGE_LOOP ( 'NONE', ( #8872, #737, #20334, #5541 ) ) ;
#8056=DIRECTION ( 'NONE',  ( 0.000000000000000000, 0.000000000000000000, -1.000000000000000000 ) ) ;
#8058=ORIENTED_EDGE ( 'NONE', *, *, #19531, .T. ) ;
#8085=FACE_OUTER_BOUND ( 'NONE', #13921, .T. ) ;
#8092=VERTEX_POINT ( 'NONE', #4572 ) ;
#8093=DIRECTION ( 'NONE',  ( 0.000000000000000000, 0.000000000000000000, 1.000000000000000000 ) ) ;
#8102=FACE_OUTER_BOUND ( 'NONE', #4925, .T. ) ;
#8103=ORIENTED_EDGE ( 'NONE', *, *, #25101, .T. ) ;
#8108=EDGE_LOOP ( 'NONE', ( #7934, #16655, #10093, #14633, #17796 ) ) ;
#8109=DIRECTION ( 'NONE',  ( -0.000000000000000000, -1.000000000000000000, -0.000000000000000000 ) ) ;
#8112=DIRECTION ( 'NONE',  ( 1.000000000000000000, 0.000000000000000000, 0.000000000000000000 ) ) ;
#8117=DIRECTION ( 'NONE',  ( -0.000000000000000000, 1.000000000000000000, -0.000000000000000000 ) ) ;
#8124=ORIENTED_EDGE ( 'NONE', *, *, #11225, .T. ) ;
#8125=CARTESIAN_POINT ( 'NONE',  ( -65.00000000000000000, -70.00000000000000000, 12.49999999999999112 ) ) ;
#8126=ORIENTED_EDGE ( 'NONE', *, *, #27842, .T. ) ;
#8130=VECTOR ( 'NONE', #24535, 1000.000000000000000 ) ;
#8138=LINE ( 'NONE', #27163, #867 ) ;
#8148=DIRECTION ( 'NONE',  ( 1.000000000000000000, 0.000000000000000000, 4.565061778886335400E-17 ) ) ;
#8152=VECTOR ( 'NONE', #17453, 1000.000000000000000 ) ;
#8157=AXIS2_PLACEMENT_3D ( 'NONE', #13139, #18582, #9367 ) ;
#8161=CARTESIAN_POINT ( 'NONE',  ( 47.00000000000044764, -4.926614671774132148E-13, 82.49999999999998579 ) ) ;
#8166=CARTESIAN_POINT ( 'NONE',  ( -50.00000000000000000, -50.00000000000000000, 62.49999999999999289 ) ) ;
#8168=DIRECTION ( 'NONE',  ( 1.000000000000000000, 0.000000000000000000, 0.000000000000000000 ) ) ;
#8178=PLANE ( 'NONE',  #30708 ) ;
#8201=FACE_OUTER_BOUND ( 'NONE', #535, .T. ) ;
#8208=EDGE_CURVE ( 'NONE', #22536, #6221, #6569, .T. ) ;
#8232=DIRECTION ( 'NONE',  ( 0.000000000000000000, 1.000000000000000000, -0.000000000000000000 ) ) ;
#8240=VERTEX_POINT ( 'NONE', #24514 ) ;
#8253=EDGE_CURVE ( 'NONE', #29075, #9580, #2174, .T. ) ;
#8260=EDGE_CURVE ( 'NONE', #7465, #24236, #12002, .T. ) ;
#8276=ORIENTED_EDGE ( 'NONE', *, *, #30149, .F. ) ;
#8282=ORIENTED_EDGE ( 'NONE', *, *, #8253, .F. ) ;
#8286=CARTESIAN_POINT ( 'NONE',  ( 37.99999999999999289, 80.00000000000000000, 0.000000000000000000 ) ) ;
#8295=AXIS2_PLACEMENT_3D ( 'NONE', #7135, #6814, #16341 ) ;
#8300=AXIS2_PLACEMENT_3D ( 'NONE', #17504, #27174, #5803 ) ;
#8303=DIRECTION ( 'NONE',  ( -1.000000000000000000, 0.000000000000000000, 0.000000000000000000 ) ) ;
#8305=PLANE ( 'NONE',  #941 ) ;
#8306=VECTOR ( 'NONE', #15013, 1000.000000000000000 ) ;
#8323=CIRCLE ( 'NONE', #3777, 29.99999999999928946 ) ;
#8324=DIRECTION ( 'NONE',  ( 1.982541115402065110E-16, 0.000000000000000000, -1.000000000000000000 ) ) ;
#8328=DIRECTION ( 'NONE',  ( 0.000000000000000000, 0.000000000000000000, -1.000000000000000000 ) ) ;
#8335=AXIS2_PLACEMENT_3D ( 'NONE', #22466, #1114, #5173 ) ;
#8345=CARTESIAN_POINT ( 'NONE',  ( 0.000000000000000000, 65.00000000000000000, 50.49999999999998579 ) ) ;
#8349=ORIENTED_EDGE ( 'NONE', *, *, #26558, .T. ) ;
#8354=AXIS2_PLACEMENT_3D ( 'NONE', #24568, #22073, #29570 ) ;
#8360=ORIENTED_EDGE ( 'NONE', *, *, #25196, .F. ) ;
#8374=FACE_OUTER_BOUND ( 'NONE', #8653, .T. ) ;
#8375=DIRECTION ( 'NONE',  ( -0.000000000000000000, 0.000000000000000000, -1.000000000000000000 ) ) ;
#8378=CARTESIAN_POINT ( 'NONE',  ( 0.000000000000000000, 87.00000000000001421, 12.49999999999999112 ) ) ;
#8380=VERTEX_POINT ( 'NONE', #21654 ) ;
#8382=FACE_BOUND ( 'NONE', #26017, .T. ) ;
#8387=AXIS2_PLACEMENT_3D ( 'NONE', #8779, #6598, #8950 ) ;
#8412=AXIS2_PLACEMENT_3D ( 'NONE', #17903, #8842, #18366 ) ;
#8424=CARTESIAN_POINT ( 'NONE',  ( 44.20394856031893482, 69.15214064669606842, 13.40394286660155210 ) ) ;
#8457=CARTESIAN_POINT ( 'NONE',  ( -37.16608720827707657, 51.86186943028246787, 97.07879600563551037 ) ) ;
#8466=CARTESIAN_POINT ( 'NONE',  ( 45.40481135428485260, 69.10336821983588607, 60.91566813060281049 ) ) ;
#8491=CARTESIAN_POINT ( 'NONE',  ( 39.99999999999998579, 63.74772708486752038, 62.49999999999999289 ) ) ;
#8499=CARTESIAN_POINT ( 'NONE',  ( -38.00000000000000000, 80.00000000000000000, 15.49999999999998579 ) ) ;
#8510=CARTESIAN_POINT ( 'NONE',  ( -2.081668171172168513E-14, 75.00000000000001421, 52.49999999999999289 ) ) ;
#8527=ORIENTED_EDGE ( 'NONE', *, *, #14985, .T. ) ;
#8528=DIRECTION ( 'NONE',  ( 0.000000000000000000, 0.000000000000000000, -1.000000000000000000 ) ) ;
#8540=DIRECTION ( 'NONE',  ( -1.000000000000000000, 0.000000000000000000, -4.565061778886335400E-17 ) ) ;
#8546=VERTEX_POINT ( 'NONE', #3567 ) ;
#8564=LINE ( 'NONE', #25398, #24542 ) ;
#8565=DIRECTION ( 'NONE',  ( -0.000000000000000000, 1.000000000000000000, 0.000000000000000000 ) ) ;
#8577=DIRECTION ( 'NONE',  ( 0.000000000000000000, 0.000000000000000000, -1.000000000000000000 ) ) ;
#8591=ORIENTED_EDGE ( 'NONE', *, *, #29583, .T. ) ;
#8600=DIRECTION ( 'NONE',  ( 0.000000000000000000, 1.000000000000000000, 0.000000000000000000 ) ) ;
#8622=AXIS2_PLACEMENT_3D ( 'NONE', #11227, #15598, #3599 ) ;
#8624=FACE_OUTER_BOUND ( 'NONE', #23936, .T. ) ;
#8629=ADVANCED_FACE ( 'NONE', ( #28358 ), #4780, .T. ) ;
#8630=PLANE ( 'NONE',  #30695 ) ;
#8635=CARTESIAN_POINT ( 'NONE',  ( 52.16608720827707657, -51.86186943028246787, 12.49999999999998401 ) ) ;
#8653=EDGE_LOOP ( 'NONE', ( #21876, #5630, #7459, #13115 ) ) ;
#8654=DIRECTION ( 'NONE',  ( 0.000000000000000000, 0.000000000000000000, 1.000000000000000000 ) ) ;
#8661=EDGE_CURVE ( 'NONE', #17425, #5751, #22986, .T. ) ;
#8675=CARTESIAN_POINT ( 'NONE',  ( 64.99999999999998579, -36.86186943028246787, 12.49999999999999112 ) ) ;
#8679=DIRECTION ( 'NONE',  ( 0.000000000000000000, 0.000000000000000000, -1.000000000000000000 ) ) ;
#8685=EDGE_LOOP ( 'NONE', ( #6679, #17449, #7672, #4338, #14178, #13565, #27908, #6271, #24480, #28066, #26208, #20426, #27777, #13212, #2311, #28326 ) ) ;
#8687=DIRECTION ( 'NONE',  ( -0.000000000000000000, -0.000000000000000000, 1.000000000000000000 ) ) ;
#8701=CARTESIAN_POINT ( 'NONE',  ( -38.00000000000000000, 80.00000000000000000, -7.533656238527846826E-15 ) ) ;
#8714=ORIENTED_EDGE ( 'NONE', *, *, #26578, .T. ) ;
#8719=CARTESIAN_POINT ( 'NONE',  ( 49.99999999999998579, 70.00000000000000000, 22.49999999999999289 ) ) ;
#8720=CARTESIAN_POINT ( 'NONE',  ( -67.00000000000000000, 50.00000000000000000, 62.49999999999999289 ) ) ;
#8733=ORIENTED_EDGE ( 'NONE', *, *, #10143, .T. ) ;
#8738=CIRCLE ( 'NONE', #754, 5.000000000000004441 ) ;
#8740=CARTESIAN_POINT ( 'NONE',  ( 39.99999999999998579, 80.00000000000001421, 22.49999999999999289 ) ) ;
#8761=VECTOR ( 'NONE', #10479, 1000.000000000000000 ) ;
#8766=VECTOR ( 'NONE', #938, 1000.000000000000000 ) ;
#8779=CARTESIAN_POINT ( 'NONE',  ( 39.99999999999998579, 87.00000000000001421, 59.49999999999999289 ) ) ;
#8793=ADVANCED_FACE ( 'NONE', ( #29619 ), #6061, .F. ) ;
#8804=ORIENTED_EDGE ( 'NONE', *, *, #13774, .T. ) ;
#8810=VECTOR ( 'NONE', #21530, 1000.000000000000000 ) ;
#8811=EDGE_CURVE ( 'NONE', #22904, #29639, #28740, .T. ) ;
#8816=ORIENTED_EDGE ( 'NONE', *, *, #21570, .T. ) ;
#8820=DIRECTION ( 'NONE',  ( -1.000000000000000000, 0.000000000000000000, 0.000000000000000000 ) ) ;
#8821=CARTESIAN_POINT ( 'NONE',  ( -42.40070334633576010, 68.50292470094652231, 12.78726508192041855 ) ) ;
#8835=FACE_OUTER_BOUND ( 'NONE', #18317, .T. ) ;
#8841=AXIS2_PLACEMENT_3D ( 'NONE', #18269, #25740, #25289 ) ;
#8842=DIRECTION ( 'NONE',  ( 0.000000000000000000, 1.000000000000000000, -0.000000000000000000 ) ) ;
#8854=CARTESIAN_POINT ( 'NONE',  ( -37.16608720827707657, 65.00000000000000000, 57.49999999999999289 ) ) ;
#8855=ORIENTED_EDGE ( 'NONE', *, *, #5206, .T. ) ;
#8872=ORIENTED_EDGE ( 'NONE', *, *, #15485, .F. ) ;
#8873=AXIS2_PLACEMENT_3D ( 'NONE', #23338, #4763, #6968 ) ;
#8885=AXIS2_PLACEMENT_3D ( 'NONE', #16172, #4163, #23485 ) ;
#8887=AXIS2_PLACEMENT_3D ( 'NONE', #18788, #20947, #4274 ) ;
#8895=CARTESIAN_POINT ( 'NONE',  ( 39.99999999999998579, 90.00000000000001421, 27.49999999999998934 ) ) ;
#8898=VERTEX_POINT ( 'NONE', #7243 ) ;
#8904=AXIS2_PLACEMENT_3D ( 'NONE', #28717, #25651, #9682 ) ;
#8906=DIRECTION ( 'NONE',  ( 0.000000000000000000, 0.000000000000000000, 1.000000000000000000 ) ) ;
#8933=CARTESIAN_POINT ( 'NONE',  ( 37.16608720827707657, 51.86186943028246787, 57.49999999999999289 ) ) ;
#8934=ORIENTED_EDGE ( 'NONE', *, *, #6189, .T. ) ;
#8937=VECTOR ( 'NONE', #27668, 1000.000000000000000 ) ;
#8939=ORIENTED_EDGE ( 'NONE', *, *, #24637, .F. ) ;
#8950=DIRECTION ( 'NONE',  ( 0.000000000000000000, 0.000000000000000000, 1.000000000000000000 ) ) ;
#8980=CARTESIAN_POINT ( 'NONE',  ( -40.58796716123164572, 67.65997107450050407, 12.49999999999998579 ) ) ;
#8987=CARTESIAN_POINT ( 'NONE',  ( 69.99999999999998579, 50.00000000000000000, 12.49999999999999112 ) ) ;
#9003=ADVANCED_FACE ( 'NONE', ( #22825 ), #22970, .T. ) ;
#9009=FACE_OUTER_BOUND ( 'NONE', #5048, .T. ) ;
#9013=VERTEX_POINT ( 'NONE', #1628 ) ;
#9018=DIRECTION ( 'NONE',  ( 0.000000000000000000, 0.000000000000000000, 1.000000000000000000 ) ) ;
#9031=EDGE_CURVE ( 'NONE', #23685, #353, #9297, .T. ) ;
#9039=DIRECTION ( 'NONE',  ( 1.000000000000000000, 0.000000000000000000, 0.000000000000000000 ) ) ;
#9041=EDGE_LOOP ( 'NONE', ( #8349, #22380 ) ) ;
#9042=EDGE_LOOP ( 'NONE', ( #25865, #15155, #4731, #24771 ) ) ;
#9051=EDGE_CURVE ( 'NONE', #14360, #28559, #9700, .T. ) ;
#9090=ORIENTED_EDGE ( 'NONE', *, *, #1998, .T. ) ;
#9102=PLANE ( 'NONE',  #30573 ) ;
#9110=ORIENTED_EDGE ( 'NONE', *, *, #5206, .F. ) ;
#9120=CARTESIAN_POINT ( 'NONE',  ( 0.000000000000000000, 0.000000000000000000, 92.49999999999998579 ) ) ;
#9121=CARTESIAN_POINT ( 'NONE',  ( -52.16608720827707657, 51.86186943028246787, 97.07879600563551037 ) ) ;
#9130=AXIS2_PLACEMENT_3D ( 'NONE', #21241, #25797, #16576 ) ;
#9131=DIRECTION ( 'NONE',  ( -1.000000000000000000, 0.000000000000000000, 0.000000000000000000 ) ) ;
#9153=DIRECTION ( 'NONE',  ( -0.000000000000000000, 1.000000000000000000, 0.000000000000000000 ) ) ;
#9164=DIRECTION ( 'NONE',  ( 0.000000000000000000, 1.000000000000000000, 0.000000000000000000 ) ) ;
#9186=AXIS2_PLACEMENT_3D ( 'NONE', #27420, #18204, #6347 ) ;
#9216=ADVANCED_FACE ( 'NONE', ( #1440, #4072 ), #6708, .F. ) ;
#9218=DIRECTION ( 'NONE',  ( 0.000000000000000000, 0.000000000000000000, 1.000000000000000000 ) ) ;
#9226=VERTEX_POINT ( 'NONE', #27480 ) ;
#9237=CARTESIAN_POINT ( 'NONE',  ( 49.99999999999998579, 50.00000000000000000, 62.49999999999999289 ) ) ;
#9239=AXIS2_PLACEMENT_3D ( 'NONE', #24926, #5899, #29609 ) ;
#9240=CYLINDRICAL_SURFACE ( 'NONE', #28725, 15.00000000000000000 ) ;
#9249=VERTEX_POINT ( 'NONE', #23079 ) ;
#9270=TOROIDAL_SURFACE ( 'NONE', #7317, 17.00000000000000000, 3.000000000000000000 ) ;
#9278=DIRECTION ( 'NONE',  ( 0.000000000000000000, 1.000000000000000000, 0.000000000000000000 ) ) ;
#9279=DIRECTION ( 'NONE',  ( -0.000000000000000000, -0.000000000000000000, -1.000000000000000000 ) ) ;
#9297=CIRCLE ( 'NONE', #14772, 10.00000000000000178 ) ;
#9301=PLANE ( 'NONE',  #30289 ) ;
#9309=( LENGTH_UNIT ( ) NAMED_UNIT ( * ) SI_UNIT ( .MILLI., .METRE. ) );
#9325=VERTEX_POINT ( 'NONE', #1589 ) ;
#9335=VECTOR ( 'NONE', #10763, 1000.000000000000000 ) ;
#9340=ORIENTED_EDGE ( 'NONE', *, *, #15862, .F. ) ;
#9347=CARTESIAN_POINT ( 'NONE',  ( 39.99999999999998579, 80.00000000000001421, 22.49999999999999289 ) ) ;
#9364=ADVANCED_FACE ( 'NONE', ( #16529 ), #9824, .F. ) ;
#9367=DIRECTION ( 'NONE',  ( 0.000000000000000000, 0.000000000000000000, -1.000000000000000000 ) ) ;
#9373=CIRCLE ( 'NONE', #24832, 5.000000000000004441 ) ;
#9389=DIRECTION ( 'NONE',  ( 1.000000000000000000, 0.000000000000000000, 4.565061778886335400E-17 ) ) ;
#9403=CARTESIAN_POINT ( 'NONE',  ( 49.99999999999998579, -50.00000000000000000, 12.49999999999999112 ) ) ;
#9423=VERTEX_POINT ( 'NONE', #29001 ) ;
#9486=CARTESIAN_POINT ( 'NONE',  ( 0.000000000000000000, 0.000000000000000000, 0.000000000000000000 ) ) ;
#9493=CIRCLE ( 'NONE', #532, 4.999999999999997335 ) ;
#9506=CIRCLE ( 'NONE', #50, 29.99999999999928946 ) ;
#9512=ORIENTED_EDGE ( 'NONE', *, *, #865, .F. ) ;
#9516=CARTESIAN_POINT ( 'NONE',  ( 52.16608720827707657, -51.86186943028246787, 57.49999999999999289 ) ) ;
#9528=CIRCLE ( 'NONE', #11036, 15.00000000000000000 ) ;
#9535=CARTESIAN_POINT ( 'NONE',  ( -7.075845757273814415E-16, 65.00000000000000000, 15.49999999999998757 ) ) ;
#9536=VECTOR ( 'NONE', #1161, 1000.000000000000000 ) ;
#9541=AXIS2_PLACEMENT_3D ( 'NONE', #13998, #9164, #14139 ) ;
#9542=LINE ( 'NONE', #16715, #16288 ) ;
#9543=EDGE_CURVE ( 'NONE', #29733, #23863, #5854, .T. ) ;
#9548=EDGE_CURVE ( 'NONE', #228, #9013, #24320, .T. ) ;
#9573=VERTEX_POINT ( 'NONE', #12486 ) ;
#9580=VERTEX_POINT ( 'NONE', #25095 ) ;
#9581=EDGE_CURVE ( 'NONE', #24152, #11965, #30073, .T. ) ;
#9582=CARTESIAN_POINT ( 'NONE',  ( 0.000000000000000000, 0.000000000000000000, 92.49999999999998579 ) ) ;
#9590=CYLINDRICAL_SURFACE ( 'NONE', #15831, 7.500000000000000000 ) ;
#9602=EDGE_CURVE ( 'NONE', #20079, #25485, #11813, .T. ) ;
#9621=VERTEX_POINT ( 'NONE', #5552 ) ;
#9648=ORIENTED_EDGE ( 'NONE', *, *, #6693, .F. ) ;
#9651=VECTOR ( 'NONE', #18070, 1000.000000000000000 ) ;
#9657=DIRECTION ( 'NONE',  ( -0.000000000000000000, 1.000000000000000000, -0.000000000000000000 ) ) ;
#9673=DIRECTION ( 'NONE',  ( -0.000000000000000000, 1.000000000000000000, 0.000000000000000000 ) ) ;
#9677=CARTESIAN_POINT ( 'NONE',  ( -67.00000000000000000, -50.00000000000000000, 62.49999999999999289 ) ) ;
#9682=DIRECTION ( 'NONE',  ( -1.000000000000000000, 0.000000000000000000, 0.000000000000000000 ) ) ;
#9688=DIRECTION ( 'NONE',  ( -1.000000000000000000, 0.000000000000000000, 0.000000000000000000 ) ) ;
#9693=ORIENTED_EDGE ( 'NONE', *, *, #4662, .T. ) ;
#9700=LINE ( 'NONE', #9860, #9811 ) ;
#9706=EDGE_CURVE ( 'NONE', #22374, #15944, #7346, .T. ) ;
#9713=ORIENTED_EDGE ( 'NONE', *, *, #9031, .F. ) ;
#9754=ORIENTED_EDGE ( 'NONE', *, *, #20037, .T. ) ;
#9789=VECTOR ( 'NONE', #5559, 1000.000000000000000 ) ;
#9803=STYLED_ITEM('',(#30879),#2927);
#9811=VECTOR ( 'NONE', #26400, 1000.000000000000000 ) ;
#9824=CYLINDRICAL_SURFACE ( 'NONE', #13323, 7.500000000000013323 ) ;
#9831=ORIENTED_EDGE ( 'NONE', *, *, #16230, .F. ) ;
#9836=ORIENTED_EDGE ( 'NONE', *, *, #18202, .T. ) ;
#9844=CIRCLE ( 'NONE', #28768, 15.00000000000000000 ) ;
#9860=CARTESIAN_POINT ( 'NONE',  ( 64.99999999999998579, -70.00000000000000000, 57.49999999999999289 ) ) ;
#9861=VECTOR ( 'NONE', #24102, 1000.000000000000000 ) ;
#9864=VECTOR ( 'NONE', #28806, 1000.000000000000000 ) ;
#9875=ORIENTED_EDGE ( 'NONE', *, *, #13975, .F. ) ;
#9878=ORIENTED_EDGE ( 'NONE', *, *, #24637, .T. ) ;
#9886=AXIS2_PLACEMENT_3D ( 'NONE', #21313, #30523, #21003 ) ;
#9889=FACE_OUTER_BOUND ( 'NONE', #24882, .T. ) ;
#9890=DIRECTION ( 'NONE',  ( 1.000000000000000000, 0.000000000000000000, 0.000000000000000000 ) ) ;
#9905=DIRECTION ( 'NONE',  ( -0.000000000000000000, 1.000000000000000000, -0.000000000000000000 ) ) ;
#9907=CARTESIAN_POINT ( 'NONE',  ( -57.50000000000001421, 50.00000000000000000, 62.49999999999999289 ) ) ;
#9913=DIRECTION ( 'NONE',  ( 0.000000000000000000, 1.000000000000000000, -0.000000000000000000 ) ) ;
#9916=DIRECTION ( 'NONE',  ( 0.000000000000000000, 0.000000000000000000, 1.000000000000000000 ) ) ;
#9918=CARTESIAN_POINT ( 'NONE',  ( -44.99999999999955236, -4.926614671774132148E-13, 82.49999999999998579 ) ) ;
#9941=DIRECTION ( 'NONE',  ( 0.000000000000000000, 0.000000000000000000, -1.000000000000000000 ) ) ;
#9945=ORIENTED_EDGE ( 'NONE', *, *, #13800, .T. ) ;
#9947=EDGE_CURVE ( 'NONE', #30435, #11497, #15167, .T. ) ;
#9949=DIRECTION ( 'NONE',  ( 0.000000000000000000, 0.000000000000000000, 1.000000000000000000 ) ) ;
#9966=ORIENTED_EDGE ( 'NONE', *, *, #15253, .T. ) ;
#9968=EDGE_CURVE ( 'NONE', #8546, #28303, #13007, .T. ) ;
#9990=LINE ( 'NONE', #4532, #11438 ) ;
#10004=EDGE_LOOP ( 'NONE', ( #22747, #22989, #16695, #270 ) ) ;
#10014=PLANE ( 'NONE',  #30186 ) ;
#10026=EDGE_CURVE ( 'NONE', #15180, #27348, #30678, .T. ) ;
#10055=LINE ( 'NONE', #5530, #6630 ) ;
#10078=PLANE ( 'NONE',  #1892 ) ;
#10093=ORIENTED_EDGE ( 'NONE', *, *, #27152, .F. ) ;
#10122=ORIENTED_EDGE ( 'NONE', *, *, #22358, .F. ) ;
#10126=CIRCLE ( 'NONE', #9130, 7.500000000000013323 ) ;
#10134=ADVANCED_FACE ( 'NONE', ( #6280 ), #3641, .F. ) ;
#10142=ORIENTED_EDGE ( 'NONE', *, *, #27792, .T. ) ;
#10143=EDGE_CURVE ( 'NONE', #14016, #4505, #26793, .T. ) ;
#10164=CARTESIAN_POINT ( 'NONE',  ( -47.14142842854255377, 69.79466010243307039, 59.50000000000029843 ) ) ;
#10180=EDGE_CURVE ( 'NONE', #20533, #6221, #27434, .T. ) ;
#10197=EDGE_CURVE ( 'NONE', #23409, #18996, #6054, .T. ) ;
#10204=LINE ( 'NONE', #5070, #27549 ) ;
#10209=CARTESIAN_POINT ( 'NONE',  ( -50.00000000000000000, -50.00000000000000000, 12.49999999999999112 ) ) ;
#10214=CARTESIAN_POINT ( 'NONE',  ( 37.16608720827707657, 65.00000000000000000, 97.07879600563551037 ) ) ;
#10217=CARTESIAN_POINT ( 'NONE',  ( 7.483314773547865784, 80.00000000000000000, 50.49999999999998579 ) ) ;
#10219=CYLINDRICAL_SURFACE ( 'NONE', #16321, 15.00000000000000000 ) ;
#10223=CARTESIAN_POINT ( 'NONE',  ( -37.16608720827707657, 65.00000000000000000, 97.07879600563551037 ) ) ;
#10225=EDGE_LOOP ( 'NONE', ( #18262, #24873, #20468, #2399 ) ) ;
#10235=VERTEX_POINT ( 'NONE', #16340 ) ;
#10246=AXIS2_PLACEMENT_3D ( 'NONE', #12422, #24560, #12726 ) ;
#10249=DIRECTION ( 'NONE',  ( 0.000000000000000000, 0.000000000000000000, 1.000000000000000000 ) ) ;
#10252=VERTEX_POINT ( 'NONE', #18675 ) ;
#10257=AXIS2_PLACEMENT_3D ( 'NONE', #18641, #6773, #8820 ) ;
#10261=LINE ( 'NONE', #28844, #6159 ) ;
#10266=EDGE_CURVE ( 'NONE', #9621, #28625, #30070, .T. ) ;
#10267=DIRECTION ( 'NONE',  ( 0.000000000000000000, -0.000000000000000000, 1.000000000000000000 ) ) ;
#10276=ORIENTED_EDGE ( 'NONE', *, *, #10523, .T. ) ;
#10278=CARTESIAN_POINT ( 'NONE',  ( 47.00000000000044764, -4.926614671774132148E-13, 79.49999999999998579 ) ) ;
#10285=AXIS2_PLACEMENT_3D ( 'NONE', #26403, #5029, #22015 ) ;
#10293=CIRCLE ( 'NONE', #2817, 15.00000000000000000 ) ;
#10312=EDGE_CURVE ( 'NONE', #16079, #5009, #26148, .T. ) ;
#10316=CARTESIAN_POINT ( 'NONE',  ( 47.14142842854284510, 69.79466010243311302, 59.49999999999998579 ) ) ;
#10317=AXIS2_PLACEMENT_3D ( 'NONE', #2088, #28462, #14569 ) ;
#10357=AXIS2_PLACEMENT_3D ( 'NONE', #1442, #30273, #20304 ) ;
#10359=ADVANCED_FACE ( 'NONE', ( #21309 ), #27401, .T. ) ;
#10363=CARTESIAN_POINT ( 'NONE',  ( -40.00000000000000000, 87.00000000000001421, 52.49999999999999289 ) ) ;
#10379=VECTOR ( 'NONE', #13711, 1000.000000000000000 ) ;
#10391=CIRCLE ( 'NONE', #8904, 7.500000000000000000 ) ;
#10401=DIRECTION ( 'NONE',  ( -0.000000000000000000, 0.000000000000000000, -1.000000000000000000 ) ) ;
#10402=PLANE ( 'NONE',  #2951 ) ;
#10404=( GEOMETRIC_REPRESENTATION_CONTEXT ( 3 ) GLOBAL_UNCERTAINTY_ASSIGNED_CONTEXT ( ( #5157 ) ) GLOBAL_UNIT_ASSIGNED_CONTEXT ( ( #433, #29741, #20384 ) ) REPRESENTATION_CONTEXT ( 'NONE', 'WORKASPACE' ) );
#10409=VERTEX_POINT ( 'NONE', #22543 ) ;
#10441=CARTESIAN_POINT ( 'NONE',  ( -42.49999999999998579, -50.00000000000000000, 12.49999999999999112 ) ) ;
#10452=CARTESIAN_POINT ( 'NONE',  ( 49.99999999999998579, 50.00000000000000000, 62.49999999999999289 ) ) ;
#10464=FACE_OUTER_BOUND ( 'NONE', #14775, .T. ) ;
#10469=LINE ( 'NONE', #29348, #14797 ) ;
#10472=DIRECTION ( 'NONE',  ( 0.000000000000000000, 0.000000000000000000, 1.000000000000000000 ) ) ;
#10475=CARTESIAN_POINT ( 'NONE',  ( 40.49651552764380114, 64.44451528374314364, 62.49999999999998579 ) ) ;
#10477=ORIENTED_EDGE ( 'NONE', *, *, #13222, .T. ) ;
#10479=DIRECTION ( 'NONE',  ( 0.000000000000000000, -1.000000000000000000, 0.000000000000000000 ) ) ;
#10484=EDGE_CURVE ( 'NONE', #9423, #12881, #14917, .T. ) ;
#10492=ORIENTED_EDGE ( 'NONE', *, *, #10545, .T. ) ;
#10498=VERTEX_POINT ( 'NONE', #29428 ) ;
#10503=EDGE_CURVE ( 'NONE', #15984, #20557, #22079, .T. ) ;
#10506=DIRECTION ( 'NONE',  ( 0.000000000000000000, 0.000000000000000000, 1.000000000000000000 ) ) ;
#10507=CARTESIAN_POINT ( 'NONE',  ( -52.16608720827707657, -36.86186943028246787, 97.07879600563551037 ) ) ;
#10523=EDGE_CURVE ( 'NONE', #26276, #6382, #26784, .T. ) ;
#10529=CARTESIAN_POINT ( 'NONE',  ( 42.49999999999998579, 50.00000000000000000, 97.07879600563551037 ) ) ;
#10539=DIRECTION ( 'NONE',  ( 0.000000000000000000, 0.000000000000000000, 1.000000000000000000 ) ) ;
#10541=FACE_OUTER_BOUND ( 'NONE', #17215, .T. ) ;
#10545=EDGE_CURVE ( 'NONE', #2627, #16462, #24426, .T. ) ;
#10577=AXIS2_PLACEMENT_3D ( 'NONE', #12870, #10827, #15337 ) ;
#10599=PLANE ( 'NONE',  #25582 ) ;
#10605=DIRECTION ( 'NONE',  ( 1.982541115402065110E-16, 0.000000000000000000, -1.000000000000000000 ) ) ;
#10607=CARTESIAN_POINT ( 'NONE',  ( 37.99999999999999289, 80.00000000000000000, 15.49999999999998934 ) ) ;
#10610=VERTEX_POINT ( 'NONE', #6324 ) ;
#10622=DIRECTION ( 'NONE',  ( 0.000000000000000000, 0.000000000000000000, -1.000000000000000000 ) ) ;
#10649=ORIENTED_EDGE ( 'NONE', *, *, #8661, .T. ) ;
#10670=EDGE_LOOP ( 'NONE', ( #3099, #18412, #23029, #3978 ) ) ;
#10679=CIRCLE ( 'NONE', #14655, 6.999999999999999112 ) ;
#10688=FACE_BOUND ( 'NONE', #21604, .T. ) ;
#10698=DIRECTION ( 'NONE',  ( -1.000000000000000000, 0.000000000000000000, -0.000000000000000000 ) ) ;
#10704=DIRECTION ( 'NONE',  ( 0.000000000000000000, 0.000000000000000000, -1.000000000000000000 ) ) ;
#10725=ORIENTED_EDGE ( 'NONE', *, *, #15262, .F. ) ;
#10728=EDGE_CURVE ( 'NONE', #11596, #24236, #19271, .T. ) ;
#10736=CARTESIAN_POINT ( 'NONE',  ( 29.99999999999925038, 1.387778780781445676E-14, 77.49999999999998579 ) ) ;
#10740=EDGE_LOOP ( 'NONE', ( #5037, #14105, #17124, #22879 ) ) ;
#10748=DIRECTION ( 'NONE',  ( -1.000000000000000000, 0.000000000000000000, 0.000000000000000000 ) ) ;
#10749=CARTESIAN_POINT ( 'NONE',  ( 4.510281037539698445E-13, -4.926614671774132148E-13, 82.49999999999998579 ) ) ;
#10750=EDGE_CURVE ( 'NONE', #18996, #19059, #14787, .T. ) ;
#10752=ORIENTED_EDGE ( 'NONE', *, *, #29770, .T. ) ;
#10759=TOROIDAL_SURFACE ( 'NONE', #13265, 7.000000000000000000, 3.000000000000000000 ) ;
#10762=VERTEX_POINT ( 'NONE', #4555 ) ;
#10763=DIRECTION ( 'NONE',  ( 1.000000000000000000, 0.000000000000000000, 0.000000000000000000 ) ) ;
#10765=EDGE_CURVE ( 'NONE', #12881, #14629, #12306, .T. ) ;
#10768=EDGE_CURVE ( 'NONE', #25063, #28591, #9542, .T. ) ;
#10772=AXIS2_PLACEMENT_3D ( 'NONE', #17462, #21659, #26505 ) ;
#10795=CARTESIAN_POINT ( 'NONE',  ( -37.99999999999933920, 4.653657836759860688E-15, 82.49999999999998579 ) ) ;
#10800=EDGE_LOOP ( 'NONE', ( #15643, #4567, #129, #17983 ) ) ;
#10806=EDGE_CURVE ( 'NONE', #3647, #15108, #13801, .T. ) ;
#10819=CARTESIAN_POINT ( 'NONE',  ( 4.510281037539698445E-13, -4.926614671774132148E-13, 57.49999999999999289 ) ) ;
#10823=AXIS2_PLACEMENT_3D ( 'NONE', #15140, #22322, #962 ) ;
#10827=DIRECTION ( 'NONE',  ( 0.000000000000000000, -1.000000000000000000, 0.000000000000000000 ) ) ;
#10853=CARTESIAN_POINT ( 'NONE',  ( -40.00000000000000000, 87.00000000000001421, 52.49999999999999289 ) ) ;
#10854=VERTEX_POINT ( 'NONE', #17336 ) ;
#10870=CARTESIAN_POINT ( 'NONE',  ( 57.49999999999998579, 50.00000000000000000, 62.49999999999999289 ) ) ;
#10871=CYLINDRICAL_SURFACE ( 'NONE', #6187, 20.00000000000000000 ) ;
#10885=EDGE_CURVE ( 'NONE', #9573, #25790, #340, .T. ) ;
#10892=CARTESIAN_POINT ( 'NONE',  ( 49.99999999999998579, -67.00000000000000000, 62.49999999999999289 ) ) ;
#10893=VERTEX_POINT ( 'NONE', #15289 ) ;
#10913=ORIENTED_EDGE ( 'NONE', *, *, #30347, .T. ) ;
#10922=EDGE_CURVE ( 'NONE', #3636, #7391, #27249, .T. ) ;
#10927=LINE ( 'NONE', #17945, #29181 ) ;
#10930=ADVANCED_FACE ( 'NONE', ( #24182 ), #10014, .F. ) ;
#10943=CARTESIAN_POINT ( 'NONE',  ( 49.99999999999998579, 50.00000000000000000, 12.49999999999999112 ) ) ;
#10964=EDGE_CURVE ( 'NONE', #13279, #20113, #25281, .T. ) ;
#10993=FACE_OUTER_BOUND ( 'NONE', #22284, .T. ) ;
#10996=DIRECTION ( 'NONE',  ( -0.000000000000000000, 1.000000000000000000, -0.000000000000000000 ) ) ;
#11011=DIRECTION ( 'NONE',  ( 0.000000000000000000, -1.000000000000000000, 0.000000000000000000 ) ) ;
#11016=DIRECTION ( 'NONE',  ( -0.000000000000000000, -0.000000000000000000, -1.000000000000000000 ) ) ;
#11018=DIRECTION ( 'NONE',  ( -1.000000000000000000, 0.000000000000000000, 0.000000000000000000 ) ) ;
#11024=DIRECTION ( 'NONE',  ( -0.000000000000000000, -0.000000000000000000, 1.000000000000000000 ) ) ;
#11026=CARTESIAN_POINT ( 'NONE',  ( -52.99999999999955236, -4.926614671774132148E-13, 62.49999999999998579 ) ) ;
#11028=ORIENTED_EDGE ( 'NONE', *, *, #12472, .F. ) ;
#11036=AXIS2_PLACEMENT_3D ( 'NONE', #11770, #9278, #1804 ) ;
#11037=DIRECTION ( 'NONE',  ( 0.000000000000000000, 1.000000000000000000, -0.000000000000000000 ) ) ;
#11040=DIRECTION ( 'NONE',  ( 0.000000000000000000, -0.000000000000000000, 1.000000000000000000 ) ) ;
#11044=ORIENTED_EDGE ( 'NONE', *, *, #10312, .F. ) ;
#11059=CARTESIAN_POINT ( 'NONE',  ( 42.39173574096481900, 68.49922546432578940, 12.78508226459883801 ) ) ;
#11092=AXIS2_PLACEMENT_3D ( 'NONE', #11948, #23465, #16461 ) ;
#11128=DIRECTION ( 'NONE',  ( -0.000000000000000000, -1.000000000000000000, -0.000000000000000000 ) ) ;
#11134=CARTESIAN_POINT ( 'NONE',  ( 52.16608720827707657, -36.86186943028246787, 12.49999999999999112 ) ) ;
#11147=LINE ( 'NONE', #23132, #19120 ) ;
#11164=LINE ( 'NONE', #3831, #7829 ) ;
#11167=CARTESIAN_POINT ( 'NONE',  ( -48.60671492705895247, 69.95510233907151587, 17.36422100552513470 ) ) ;
#11170=CARTESIAN_POINT ( 'NONE',  ( 49.99999999999998579, 70.00000000000000000, 12.49999999999999112 ) ) ;
#11173=PLANE ( 'NONE',  #124 ) ;
#11183=CARTESIAN_POINT ( 'NONE',  ( 37.16608720827707657, 36.86186943028246787, 57.49999999999999289 ) ) ;
#11194=EDGE_CURVE ( 'NONE', #27603, #23407, #1252, .T. ) ;
#11195=VECTOR ( 'NONE', #28786, 1000.000000000000000 ) ;
#11211=ORIENTED_EDGE ( 'NONE', *, *, #15638, .F. ) ;
#11216=ORIENTED_EDGE ( 'NONE', *, *, #18202, .F. ) ;
#11225=EDGE_CURVE ( 'NONE', #12499, #27312, #17736, .T. ) ;
#11227=CARTESIAN_POINT ( 'NONE',  ( 39.99999999999998579, 87.00000000000001421, 22.49999999999999289 ) ) ;
#11268=EDGE_CURVE ( 'NONE', #4505, #25524, #10927, .T. ) ;
#11271=DIRECTION ( 'NONE',  ( -1.000000000000000000, 0.000000000000000000, 0.000000000000000000 ) ) ;
#11277=VERTEX_POINT ( 'NONE', #10607 ) ;
#11281=EDGE_LOOP ( 'NONE', ( #4604, #15230, #8934, #10477 ) ) ;
#11303=EDGE_CURVE ( 'NONE', #8240, #8380, #2158, .T. ) ;
#11340=ADVANCED_FACE ( 'NONE', ( #6834 ), #27916, .F. ) ;
#11341=AXIS2_PLACEMENT_3D ( 'NONE', #26777, #12898, #6015 ) ;
#11344=CIRCLE ( 'NONE', #3360, 5.000000000000004441 ) ;
#11381=CARTESIAN_POINT ( 'NONE',  ( 4.510281037539698445E-13, -4.926614671774132148E-13, 82.49999999999998579 ) ) ;
#11385=ORIENTED_EDGE ( 'NONE', *, *, #232, .T. ) ;
#11394=CARTESIAN_POINT ( 'NONE',  ( -40.00000000000002842, 80.00000000000001421, 22.49999999999983302 ) ) ;
#11413=AXIS2_PLACEMENT_3D ( 'NONE', #2577, #5069, #11947 ) ;
#11421=DIRECTION ( 'NONE',  ( -1.000000000000000000, 0.000000000000000000, 0.000000000000000000 ) ) ;
#11424=LINE ( 'NONE', #30436, #21777 ) ;
#11434=CARTESIAN_POINT ( 'NONE',  ( -52.99999999999955236, -4.926614671774132148E-13, 65.49999999999998579 ) ) ;
#11438=VECTOR ( 'NONE', #2652, 1000.000000000000000 ) ;
#11446=AXIS2_PLACEMENT_3D ( 'NONE', #25911, #4390, #23250 ) ;
#11448=ORIENTED_EDGE ( 'NONE', *, *, #10768, .F. ) ;
#11462=ORIENTED_EDGE ( 'NONE', *, *, #29004, .F. ) ;
#11464=ADVANCED_FACE ( 'NONE', ( #13716 ), #27763, .T. ) ;
#11467=DIRECTION ( 'NONE',  ( 0.000000000000000000, -0.000000000000000000, -1.000000000000000000 ) ) ;
#11474=CARTESIAN_POINT ( 'NONE',  ( -49.32716953814647809, 69.98911764784745060, 18.87824250137748550 ) ) ;
#11497=VERTEX_POINT ( 'NONE', #13076 ) ;
#11525=ADVANCED_FACE ( 'NONE', ( #8085 ), #731, .F. ) ;
#11530=CIRCLE ( 'NONE', #2549, 7.500000000000000000 ) ;
#11538=CARTESIAN_POINT ( 'NONE',  ( 4.510281037539698445E-13, -4.926614671774132148E-13, 79.49999999999998579 ) ) ;
#11542=ADVANCED_FACE ( 'NONE', ( #24751 ), #5436, .T. ) ;
#11561=LINE ( 'NONE', #6264, #20884 ) ;
#11566=CARTESIAN_POINT ( 'NONE',  ( 0.000000000000000000, 0.000000000000000000, 85.49999999999998579 ) ) ;
#11573=CIRCLE ( 'NONE', #26514, 10.00000000000000178 ) ;
#11596=VERTEX_POINT ( 'NONE', #21415 ) ;
#11611=VECTOR ( 'NONE', #19619, 1000.000000000000000 ) ;
#11626=DIRECTION ( 'NONE',  ( 0.000000000000000000, 0.000000000000000000, -1.000000000000000000 ) ) ;
#11628=ORIENTED_EDGE ( 'NONE', *, *, #18135, .F. ) ;
#11637=AXIS2_PLACEMENT_3D ( 'NONE', #22334, #29515, #3776 ) ;
#11642=VERTEX_POINT ( 'NONE', #20394 ) ;
#11656=DIRECTION ( 'NONE',  ( -1.000000000000000000, 0.000000000000000000, 0.000000000000000000 ) ) ;
#11657=CIRCLE ( 'NONE', #15639, 7.500000000000013323 ) ;
#11668=CARTESIAN_POINT ( 'NONE',  ( -50.00000000000000711, 70.00000000000001421, 53.15210795805025867 ) ) ;
#11670=ORIENTED_EDGE ( 'NONE', *, *, #9581, .T. ) ;
#11671=DIRECTION ( 'NONE',  ( 1.000000000000000000, 0.000000000000000000, 0.000000000000000000 ) ) ;
#11678=ADVANCED_FACE ( 'NONE', ( #6926 ), #14231, .T. ) ;
#11680=DIRECTION ( 'NONE',  ( 0.000000000000000000, -0.000000000000000000, 1.000000000000000000 ) ) ;
#11692=ORIENTED_EDGE ( 'NONE', *, *, #17924, .T. ) ;
#11712=CARTESIAN_POINT ( 'NONE',  ( 49.99999999999998579, -50.00000000000000000, 97.07879600563551037 ) ) ;
#11752=ORIENTED_EDGE ( 'NONE', *, *, #10026, .T. ) ;
#11758=DIRECTION ( 'NONE',  ( 0.000000000000000000, 0.000000000000000000, 1.000000000000000000 ) ) ;
#11770=CARTESIAN_POINT ( 'NONE',  ( -2.081668171172168513E-14, 90.00000000000001421, 37.49999999999999289 ) ) ;
#11787=ORIENTED_EDGE ( 'NONE', *, *, #13724, .F. ) ;
#11789=VECTOR ( 'NONE', #20201, 1000.000000000000000 ) ;
#11807=AXIS2_PLACEMENT_3D ( 'NONE', #22397, #22235, #13048 ) ;
#11810=CARTESIAN_POINT ( 'NONE',  ( -64.99999999999998579, 36.86186943028246787, 97.07879600563551037 ) ) ;
#11813=CIRCLE ( 'NONE', #29255, 20.00000000000000000 ) ;
#11814=LINE ( 'NONE', #114, #15058 ) ;
#11815=EDGE_LOOP ( 'NONE', ( #3809, #24646, #19761, #22558 ) ) ;
#11823=AXIS2_PLACEMENT_3D ( 'NONE', #9403, #28893, #26549 ) ;
#11829=ADVANCED_FACE ( 'NONE', ( #12692 ), #19244, .T. ) ;
#11844=DIRECTION ( 'NONE',  ( 0.000000000000000000, 0.000000000000000000, 1.000000000000000000 ) ) ;
#11845=AXIS2_PLACEMENT_3D ( 'NONE', #25284, #13451, #18265 ) ;
#11853=CARTESIAN_POINT ( 'NONE',  ( -50.00000000000000000, 50.00000000000000000, 62.49999999999999289 ) ) ;
#11895=ADVANCED_FACE ( 'NONE', ( #8624 ), #29991, .F. ) ;
#11896=DIRECTION ( 'NONE',  ( 0.000000000000000000, 1.000000000000000000, 0.000000000000000000 ) ) ;
#11916=ORIENTED_EDGE ( 'NONE', *, *, #1608, .F. ) ;
#11947=DIRECTION ( 'NONE',  ( 0.000000000000000000, 0.000000000000000000, 1.000000000000000000 ) ) ;
#11948=CARTESIAN_POINT ( 'NONE',  ( -67.00000000000000000, -50.00000000000000000, 59.49999999999999289 ) ) ;
#11965=VERTEX_POINT ( 'NONE', #12847 ) ;
#12001=DIRECTION ( 'NONE',  ( -1.000000000000000000, 0.000000000000000000, 0.000000000000000000 ) ) ;
#12002=LINE ( 'NONE', #4817, #1094 ) ;
#12033=ORIENTED_EDGE ( 'NONE', *, *, #27367, .T. ) ;
#12056=EDGE_CURVE ( 'NONE', #10498, #21378, #19409, .T. ) ;
#12058=LINE ( 'NONE', #14393, #5435 ) ;
#12084=DIRECTION ( 'NONE',  ( 0.000000000000000000, -0.000000000000000000, 1.000000000000000000 ) ) ;
#12099=CARTESIAN_POINT ( 'NONE',  ( -29.99999999999933209, 1.755172820525642916E-14, 67.49999999999997158 ) ) ;
#12119=ORIENTED_EDGE ( 'NONE', *, *, #2901, .F. ) ;
#12120=DIRECTION ( 'NONE',  ( 0.000000000000000000, -1.000000000000000000, 0.000000000000000000 ) ) ;
#12138=ORIENTED_EDGE ( 'NONE', *, *, #12602, .T. ) ;
#12162=CARTESIAN_POINT ( 'NONE',  ( -70.00000000000000000, -65.00000000000000000, 12.49999999999999112 ) ) ;
#12166=LINE ( 'NONE', #14501, #15098 ) ;
#12184=ORIENTED_EDGE ( 'NONE', *, *, #10922, .F. ) ;
#12187=ORIENTED_EDGE ( 'NONE', *, *, #23091, .T. ) ;
#12193=CARTESIAN_POINT ( 'NONE',  ( -40.00000000000002842, 90.00000000000001421, 22.49999999999983302 ) ) ;
#12207=DIRECTION ( 'NONE',  ( 0.000000000000000000, 0.000000000000000000, 1.000000000000000000 ) ) ;
#12234=DIRECTION ( 'NONE',  ( -1.000000000000000000, 0.000000000000000000, 0.000000000000000000 ) ) ;
#12241=ORIENTED_EDGE ( 'NONE', *, *, #13222, .F. ) ;
#12248=ORIENTED_EDGE ( 'NONE', *, *, #29224, .F. ) ;
#12261=VERTEX_POINT ( 'NONE', #8895 ) ;
#12262=ADVANCED_FACE ( 'NONE', ( #6840 ), #18419, .F. ) ;
#12281=ADVANCED_FACE ( 'NONE', ( #4198 ), #25869, .T. ) ;
#12285=VERTEX_POINT ( 'NONE', #18558 ) ;
#12297=TOROIDAL_SURFACE ( 'NONE', #16277, 17.00000000000000000, 3.000000000000000000 ) ;
#12302=CIRCLE ( 'NONE', #24806, 53.00000000000000711 ) ;
#12306=CIRCLE ( 'NONE', #17792, 15.00000000000000000 ) ;
#12319=AXIS2_PLACEMENT_3D ( 'NONE', #14612, #24114, #7447 ) ;
#12350=PLANE ( 'NONE',  #6360 ) ;
#12351=CARTESIAN_POINT ( 'NONE',  ( 0.000000000000000000, 87.00000000000001421, 59.49999999999999289 ) ) ;
#12362=CARTESIAN_POINT ( 'NONE',  ( -40.00000000000000711, 87.00000000000001421, 62.49999999999999289 ) ) ;
#12363=DIRECTION ( 'NONE',  ( -0.000000000000000000, -0.000000000000000000, 1.000000000000000000 ) ) ;
#12367=AXIS2_PLACEMENT_3D ( 'NONE', #22119, #17135, #10267 ) ;
#12370=CARTESIAN_POINT ( 'NONE',  ( 4.510281037539698445E-13, -4.926614671774132148E-13, 57.49999999999999289 ) ) ;
#12371=ORIENTED_EDGE ( 'NONE', *, *, #8253, .T. ) ;
#12393=DIRECTION ( 'NONE',  ( 0.000000000000000000, 1.000000000000000000, -0.000000000000000000 ) ) ;
#12397=EDGE_LOOP ( 'NONE', ( #22881, #26359 ) ) ;
#12402=LINE ( 'NONE', #2574, #7307 ) ;
#12415=SHAPE_DEFINITION_REPRESENTATION ( #14407, #13696 ) ;
#12422=CARTESIAN_POINT ( 'NONE',  ( -37.16608720827707657, -36.86186943028246787, 97.07879600563551037 ) ) ;
#12429=AXIS2_PLACEMENT_3D ( 'NONE', #11538, #25428, #2164 ) ;
#12438=ADVANCED_FACE ( 'NONE', ( #27560 ), #13950, .F. ) ;
#12443=DIRECTION ( 'NONE',  ( -0.000000000000000000, 1.000000000000000000, -0.000000000000000000 ) ) ;
#12445=ORIENTED_EDGE ( 'NONE', *, *, #12460, .F. ) ;
#12452=EDGE_CURVE ( 'NONE', #9573, #228, #24742, .T. ) ;
#12453=LINE ( 'NONE', #17579, #1684 ) ;
#12460=EDGE_CURVE ( 'NONE', #19119, #23409, #26405, .T. ) ;
#12472=EDGE_CURVE ( 'NONE', #886, #27348, #22896, .T. ) ;
#12480=ORIENTED_EDGE ( 'NONE', *, *, #9543, .F. ) ;
#12486=CARTESIAN_POINT ( 'NONE',  ( -35.41742430504425698, 80.00000000000001421, 50.49999999999998579 ) ) ;
#12490=AXIS2_PLACEMENT_3D ( 'NONE', #2784, #8232, #29601 ) ;
#12491=FACE_OUTER_BOUND ( 'NONE', #10740, .T. ) ;
#12499=VERTEX_POINT ( 'NONE', #10870 ) ;
#12502=ADVANCED_FACE ( 'NONE', ( #25371, #27246, #8382, #4001, #20069, #23009 ), #15213, .T. ) ;
#12504=DIRECTION ( 'NONE',  ( 1.000000000000000000, 0.000000000000000000, 0.000000000000000000 ) ) ;
#12517=DIRECTION ( 'NONE',  ( 1.000000000000000000, 0.000000000000000000, -0.000000000000000000 ) ) ;
#12523=FACE_OUTER_BOUND ( 'NONE', #3202, .T. ) ;
#12531=ORIENTED_EDGE ( 'NONE', *, *, #4260, .T. ) ;
#12537=CARTESIAN_POINT ( 'NONE',  ( -40.00000000000000000, 87.00000000000001421, 22.49999999999999289 ) ) ;
#12540=ORIENTED_EDGE ( 'NONE', *, *, #412, .T. ) ;
#12543=FACE_OUTER_BOUND ( 'NONE', #19998, .T. ) ;
#12555=DIRECTION ( 'NONE',  ( 0.000000000000000000, 0.000000000000000000, -1.000000000000000000 ) ) ;
#12586=FACE_OUTER_BOUND ( 'NONE', #28498, .T. ) ;
#12602=EDGE_CURVE ( 'NONE', #20557, #16079, #16157, .T. ) ;
#12615=ADVANCED_FACE ( 'NONE', ( #4606 ), #3986, .T. ) ;
#12647=VECTOR ( 'NONE', #13810, 1000.000000000000000 ) ;
#12660=ORIENTED_EDGE ( 'NONE', *, *, #29964, .F. ) ;
#12692=FACE_OUTER_BOUND ( 'NONE', #14819, .T. ) ;
#12693=ORIENTED_EDGE ( 'NONE', *, *, #27295, .T. ) ;
#12707=ORIENTED_EDGE ( 'NONE', *, *, #13569, .T. ) ;
#12714=ORIENTED_EDGE ( 'NONE', *, *, #2134, .T. ) ;
#12726=DIRECTION ( 'NONE',  ( 0.000000000000000000, -0.000000000000000000, 1.000000000000000000 ) ) ;
#12729=VERTEX_POINT ( 'NONE', #5073 ) ;
#12739=CARTESIAN_POINT ( 'NONE',  ( 37.99999999999999289, 65.00000000000000000, -0.000000000000000000 ) ) ;
#12742=CARTESIAN_POINT ( 'NONE',  ( 49.99999999999998579, -50.00000000000000000, 12.49999999999999112 ) ) ;
#12754=AXIS2_PLACEMENT_3D ( 'NONE', #5397, #26613, #9916 ) ;
#12755=ORIENTED_EDGE ( 'NONE', *, *, #4988, .T. ) ;
#12762=VERTEX_POINT ( 'NONE', #3042 ) ;
#12775=CARTESIAN_POINT ( 'NONE',  ( -37.16608720827707657, -65.00000000000000000, 57.49999999999999289 ) ) ;
#12785=ORIENTED_EDGE ( 'NONE', *, *, #3472, .T. ) ;
#12789=DIRECTION ( 'NONE',  ( 0.000000000000000000, -1.000000000000000000, 0.000000000000000000 ) ) ;
#12793=LINE ( 'NONE', #13106, #3219 ) ;
#12801=VERTEX_POINT ( 'NONE', #14888 ) ;
#12825=VERTEX_POINT ( 'NONE', #12099 ) ;
#12840=VECTOR ( 'NONE', #25628, 1000.000000000000000 ) ;
#12847=CARTESIAN_POINT ( 'NONE',  ( 49.99999999999998579, 70.00000000000000000, 22.49999999999999289 ) ) ;
#12849=ORIENTED_EDGE ( 'NONE', *, *, #26444, .F. ) ;
#12862=EDGE_CURVE ( 'NONE', #353, #24053, #1316, .T. ) ;
#12870=CARTESIAN_POINT ( 'NONE',  ( -40.00000000000000000, 0.000000000000000000, 52.49999999999999289 ) ) ;
#12881=VERTEX_POINT ( 'NONE', #20343 ) ;
#12887=AXIS2_PLACEMENT_3D ( 'NONE', #14713, #4738, #14570 ) ;
#12891=ORIENTED_EDGE ( 'NONE', *, *, #29834, .T. ) ;
#12894=DIRECTION ( 'NONE',  ( 0.000000000000000000, 1.000000000000000000, 0.000000000000000000 ) ) ;
#12898=DIRECTION ( 'NONE',  ( -1.000000000000000000, 0.000000000000000000, 0.000000000000000000 ) ) ;
#12910=DIRECTION ( 'NONE',  ( -1.000000000000000000, 0.000000000000000000, 0.000000000000000000 ) ) ;
#12915=DIRECTION ( 'NONE',  ( -1.000000000000000000, 0.000000000000000000, -0.000000000000000000 ) ) ;
#12918=CIRCLE ( 'NONE', #19359, 20.00000000000000000 ) ;
#12925=CARTESIAN_POINT ( 'NONE',  ( 0.000000000000000000, -67.00000000000000000, 59.49999999999999289 ) ) ;
#12933=CARTESIAN_POINT ( 'NONE',  ( -40.00000000000002842, 90.00000000000001421, 52.50000000000014921 ) ) ;
#12935=LINE ( 'NONE', #15236, #9651 ) ;
#12939=DIRECTION ( 'NONE',  ( -0.000000000000000000, -0.000000000000000000, -1.000000000000000000 ) ) ;
#12950=ORIENTED_EDGE ( 'NONE', *, *, #16117, .T. ) ;
#12963=AXIS2_PLACEMENT_3D ( 'NONE', #15851, #8687, #1663 ) ;
#12965=ADVANCED_FACE ( 'NONE', ( #10993 ), #5998, .F. ) ;
#12967=EDGE_CURVE ( 'NONE', #24377, #26649, #25331, .T. ) ;
#12982=CARTESIAN_POINT ( 'NONE',  ( -42.73636061667930619, 67.00059800727392201, 62.14018330172965676 ) ) ;
#12985=FACE_OUTER_BOUND ( 'NONE', #3250, .T. ) ;
#12988=ORIENTED_EDGE ( 'NONE', *, *, #18687, .T. ) ;
#12994=EDGE_CURVE ( 'NONE', #5751, #3636, #17691, .T. ) ;
#12995=ORIENTED_EDGE ( 'NONE', *, *, #27856, .T. ) ;
#13007=LINE ( 'NONE', #22497, #17312 ) ;
#13012=EDGE_CURVE ( 'NONE', #6382, #15984, #29701, .T. ) ;
#13015=DIRECTION ( 'NONE',  ( 0.000000000000000000, -0.000000000000000000, -1.000000000000000000 ) ) ;
#13043=DIRECTION ( 'NONE',  ( 0.000000000000000000, 0.000000000000000000, 1.000000000000000000 ) ) ;
#13047=ORIENTED_EDGE ( 'NONE', *, *, #4662, .F. ) ;
#13048=DIRECTION ( 'NONE',  ( 0.000000000000000000, 0.000000000000000000, 1.000000000000000000 ) ) ;
#13052=DIRECTION ( 'NONE',  ( 1.000000000000000000, 0.000000000000000000, 0.000000000000000000 ) ) ;
#13067=CARTESIAN_POINT ( 'NONE',  ( -50.00000000000000000, -70.00000000000000000, 59.49999999999999289 ) ) ;
#13070=CIRCLE ( 'NONE', #30471, 4.999999999999997335 ) ;
#13076=CARTESIAN_POINT ( 'NONE',  ( 39.99999999999998579, 90.00000000000001421, 47.49999999999999289 ) ) ;
#13078=FACE_BOUND ( 'NONE', #22985, .T. ) ;
#13096=CARTESIAN_POINT ( 'NONE',  ( 39.99999999999998579, 90.00000000000001421, 15.49999999999999289 ) ) ;
#13099=CARTESIAN_POINT ( 'NONE',  ( 46.42112861060978446, 69.67901318393784038, 14.82662894843562107 ) ) ;
#13106=CARTESIAN_POINT ( 'NONE',  ( 50.00000000000045475, -4.865382331816764069E-13, 82.49999999999998579 ) ) ;
#13115=ORIENTED_EDGE ( 'NONE', *, *, #4928, .F. ) ;
#13120=CIRCLE ( 'NONE', #655, 15.00000000000000000 ) ;
#13131=CARTESIAN_POINT ( 'NONE',  ( 45.88720470728337375, 69.36824064663011313, 60.58574961613483367 ) ) ;
#13139=CARTESIAN_POINT ( 'NONE',  ( 39.99999999999998579, 80.00000000000001421, 52.49999999999999289 ) ) ;
#13141=CIRCLE ( 'NONE', #20576, 3.000000000000002665 ) ;
#13148=ORIENTED_EDGE ( 'NONE', *, *, #14699, .F. ) ;
#13150=DIRECTION ( 'NONE',  ( 0.000000000000000000, -1.000000000000000000, 0.000000000000000000 ) ) ;
#13168=DIRECTION ( 'NONE',  ( 0.000000000000000000, 0.000000000000000000, -1.000000000000000000 ) ) ;
#13194=CARTESIAN_POINT ( 'NONE',  ( -37.16608720827707657, 65.00000000000000000, 12.49999999999999112 ) ) ;
#13210=ORIENTED_EDGE ( 'NONE', *, *, #26439, .T. ) ;
#13212=ORIENTED_EDGE ( 'NONE', *, *, #30546, .T. ) ;
#13222=EDGE_CURVE ( 'NONE', #2571, #15921, #12058, .T. ) ;
#13223=ORIENTED_EDGE ( 'NONE', *, *, #17404, .T. ) ;
#13224=ORIENTED_EDGE ( 'NONE', *, *, #16230, .T. ) ;
#13235=DIRECTION ( 'NONE',  ( 0.000000000000000000, 0.000000000000000000, -1.000000000000000000 ) ) ;
#13255=CARTESIAN_POINT ( 'NONE',  ( 45.62014130220955366, 69.51663404683095848, 14.22215358659609130 ) ) ;
#13265=AXIS2_PLACEMENT_3D ( 'NONE', #30338, #25514, #4136 ) ;
#13278=CARTESIAN_POINT ( 'NONE',  ( -40.00000000000000000, 87.00000000000001421, 22.49999999999999289 ) ) ;
#13279=VERTEX_POINT ( 'NONE', #3619 ) ;
#13292=CIRCLE ( 'NONE', #16763, 15.00000000000000000 ) ;
#13313=CARTESIAN_POINT ( 'NONE',  ( -38.00000000000000000, 80.00000000000000000, -7.533656238527846826E-15 ) ) ;
#13314=CARTESIAN_POINT ( 'NONE',  ( 37.16608720827707657, 65.00000000000000000, 97.07879600563551037 ) ) ;
#13318=VECTOR ( 'NONE', #12120, 1000.000000000000000 ) ;
#13323=AXIS2_PLACEMENT_3D ( 'NONE', #445, #14181, #2646 ) ;
#13343=ORIENTED_EDGE ( 'NONE', *, *, #22555, .F. ) ;
#13359=CARTESIAN_POINT ( 'NONE',  ( -42.09461541023539155, 68.37430988400880949, 12.71698366717900619 ) ) ;
#13363=DIRECTION ( 'NONE',  ( 1.000000000000000000, 0.000000000000000000, 0.000000000000000000 ) ) ;
#13369=ORIENTED_EDGE ( 'NONE', *, *, #7480, .F. ) ;
#13372=DIRECTION ( 'NONE',  ( -1.000000000000000000, 0.000000000000000000, 0.000000000000000000 ) ) ;
#13399=DIRECTION ( 'NONE',  ( 0.000000000000000000, 0.000000000000000000, -1.000000000000000000 ) ) ;
#13400=B_SPLINE_CURVE_WITH_KNOTS ( 'NONE', 3,
 ( #20298, #10475, #24659, #5956, #15454, #15292, #7996, #24822, #19988, #8466, #24972, #13131, #22010, #22625, #794, #10316 ),
 .UNSPECIFIED., .F., .F.,
 ( 4, 2, 2, 2, 2, 2, 2, 4 ),
 ( -2.365086329950664848E-05, 0.002543131582615900527, 0.005109914028531307648, 0.006393305251489012943, 0.007676696474446719105, 0.008318392085925573054, 0.008960087697404424401, 0.01024347892036214444 ),
 .UNSPECIFIED. ) ;
#13416=EDGE_LOOP ( 'NONE', ( #2030, #9713, #19202, #27137 ) ) ;
#13419=CARTESIAN_POINT ( 'NONE',  ( 40.58772298843799575, 67.65983010127237662, 12.49999999999999289 ) ) ;
#13424=CARTESIAN_POINT ( 'NONE',  ( -40.00000000000002842, 80.00000000000001421, 27.49999999999983658 ) ) ;
#13433=ADVANCED_FACE ( 'NONE', ( #22176, #29667 ), #8305, .T. ) ;
#13451=DIRECTION ( 'NONE',  ( 0.000000000000000000, 1.000000000000000000, 0.000000000000000000 ) ) ;
#13466=EDGE_CURVE ( 'NONE', #12285, #8898, #1598, .T. ) ;
#13474=DIRECTION ( 'NONE',  ( -1.000000000000000000, 0.000000000000000000, 0.000000000000000000 ) ) ;
#13475=EDGE_LOOP ( 'NONE', ( #4083, #12445, #13954, #29456 ) ) ;
#13490=DIRECTION ( 'NONE',  ( -1.000000000000000000, 0.000000000000000000, 0.000000000000000000 ) ) ;
#13502=CARTESIAN_POINT ( 'NONE',  ( -15.00000000000004086, 1.571475800653548713E-14, 92.49999999999998579 ) ) ;
#13504=ORIENTED_EDGE ( 'NONE', *, *, #30184, .T. ) ;
#13561=ORIENTED_EDGE ( 'NONE', *, *, #27792, .F. ) ;
#13564=DIRECTION ( 'NONE',  ( 1.000000000000000000, 0.000000000000000000, 0.000000000000000000 ) ) ;
#13565=ORIENTED_EDGE ( 'NONE', *, *, #30149, .T. ) ;
#13569=EDGE_CURVE ( 'NONE', #28974, #9226, #23692, .T. ) ;
#13618=CYLINDRICAL_SURFACE ( 'NONE', #24758, 7.500000000000013323 ) ;
#13619=AXIS2_PLACEMENT_3D ( 'NONE', #16029, #7556, #25854 ) ;
#13623=AXIS2_PLACEMENT_3D ( 'NONE', #16423, #18616, #27976 ) ;
#13632=CARTESIAN_POINT ( 'NONE',  ( 49.99999999999998579, 90.00000000000001421, 52.49999999999999289 ) ) ;
#13643=CIRCLE ( 'NONE', #28070, 15.00000000000000000 ) ;
#13649=CARTESIAN_POINT ( 'NONE',  ( 69.99999999999998579, 50.00000000000000000, 12.49999999999999112 ) ) ;
#13664=ORIENTED_EDGE ( 'NONE', *, *, #15307, .T. ) ;
#13671=CARTESIAN_POINT ( 'NONE',  ( 0.000000000000000000, 0.000000000000000000, 92.49999999999998579 ) ) ;
#13695=ORIENTED_EDGE ( 'NONE', *, *, #14508, .F. ) ;
#13696=SHAPE_REPRESENTATION ( 'Housing  Cover Cap', ( #7396 ), #10404 ) ;
#13711=DIRECTION ( 'NONE',  ( 0.000000000000000000, 0.000000000000000000, -1.000000000000000000 ) ) ;
#13714=PLANE ( 'NONE',  #26372 ) ;
#13716=FACE_OUTER_BOUND ( 'NONE', #22421, .T. ) ;
#13724=EDGE_CURVE ( 'NONE', #24236, #11596, #21839, .T. ) ;
#13737=ORIENTED_EDGE ( 'NONE', *, *, #17549, .T. ) ;
#13742=CARTESIAN_POINT ( 'NONE',  ( 39.99999999999998579, 80.00000000000001421, 47.49999999999999289 ) ) ;
#13749=CYLINDRICAL_SURFACE ( 'NONE', #22184, 7.500000000000000000 ) ;
#13751=ORIENTED_EDGE ( 'NONE', *, *, #29759, .F. ) ;
#13752=CIRCLE ( 'NONE', #17729, 3.000000000000002665 ) ;
#13765=CARTESIAN_POINT ( 'NONE',  ( 39.99999999999998579, 80.00000000000001421, 52.49999999999999289 ) ) ;
#13767=DIRECTION ( 'NONE',  ( -1.000000000000000000, 0.000000000000000000, 0.000000000000000000 ) ) ;
#13774=EDGE_CURVE ( 'NONE', #15313, #23863, #15399, .T. ) ;
#13785=EDGE_CURVE ( 'NONE', #11965, #353, #14895, .T. ) ;
#13790=CARTESIAN_POINT ( 'NONE',  ( 37.16608720827707657, -51.86186943028246787, 12.49999999999999112 ) ) ;
#13800=EDGE_CURVE ( 'NONE', #25790, #25448, #19891, .T. ) ;
#13801=CIRCLE ( 'NONE', #10823, 29.99999999999928946 ) ;
#13803=CARTESIAN_POINT ( 'NONE',  ( 39.99999999999998579, 80.00000000000001421, 52.49999999999999289 ) ) ;
#13810=DIRECTION ( 'NONE',  ( 0.000000000000000000, 0.000000000000000000, -1.000000000000000000 ) ) ;
#13811=CARTESIAN_POINT ( 'NONE',  ( -47.38851077911648702, 69.82999317555587027, 15.75289764418246286 ) ) ;
#13816=DIRECTION ( 'NONE',  ( 0.000000000000000000, 0.000000000000000000, -1.000000000000000000 ) ) ;
#13824=DIRECTION ( 'NONE',  ( -1.000000000000000000, 0.000000000000000000, 0.000000000000000000 ) ) ;
#13846=EDGE_LOOP ( 'NONE', ( #1433, #3605, #6407, #9831 ) ) ;
#13850=DIRECTION ( 'NONE',  ( -1.000000000000000000, 0.000000000000000000, 0.000000000000000000 ) ) ;
#13857=AXIS2_PLACEMENT_3D ( 'NONE', #28668, #7148, #6678 ) ;
#13890=ORIENTED_EDGE ( 'NONE', *, *, #17549, .F. ) ;
#13892=PRODUCT_DEFINITION_FORMATION_WITH_SPECIFIED_SOURCE ( 'ANY', '', #7963, .NOT_KNOWN. ) ;
#13893=DIRECTION ( 'NONE',  ( 0.000000000000000000, 1.000000000000000000, 0.000000000000000000 ) ) ;
#13903=CARTESIAN_POINT ( 'NONE',  ( -40.00000000000002842, 80.00000000000001421, 52.50000000000014921 ) ) ;
#13906=CARTESIAN_POINT ( 'NONE',  ( 37.99999999999999289, 80.00000000000001421, 17.91742430504415040 ) ) ;
#13921=EDGE_LOOP ( 'NONE', ( #4225, #5004, #18110, #30116 ) ) ;
#13950=TOROIDAL_SURFACE ( 'NONE', #5476, 53.00000000000000711, 3.000000000000000000 ) ;
#13951=PLANE ( 'NONE',  #6862 ) ;
#13954=ORIENTED_EDGE ( 'NONE', *, *, #23339, .F. ) ;
#13975=EDGE_CURVE ( 'NONE', #21378, #10498, #10126, .T. ) ;
#13988=FACE_OUTER_BOUND ( 'NONE', #24958, .T. ) ;
#13998=CARTESIAN_POINT ( 'NONE',  ( 39.99999999999998579, 90.00000000000001421, 22.49999999999999289 ) ) ;
#14007=ORIENTED_EDGE ( 'NONE', *, *, #201, .T. ) ;
#14016=VERTEX_POINT ( 'NONE', #13790 ) ;
#14039=CARTESIAN_POINT ( 'NONE',  ( -4.163336342344337027E-14, 1.387778780781445676E-14, 67.49999999999997158 ) ) ;
#14046=DIRECTION ( 'NONE',  ( -0.000000000000000000, -0.000000000000000000, 1.000000000000000000 ) ) ;
#14061=CARTESIAN_POINT ( 'NONE',  ( 37.99999999999999289, 80.00000000000001421, 50.49999999999998579 ) ) ;
#14100=FACE_OUTER_BOUND ( 'NONE', #24451, .T. ) ;
#14105=ORIENTED_EDGE ( 'NONE', *, *, #26558, .F. ) ;
#14107=DIRECTION ( 'NONE',  ( 0.000000000000000000, 0.000000000000000000, -1.000000000000000000 ) ) ;
#14117=EDGE_CURVE ( 'NONE', #3636, #24493, #19149, .T. ) ;
#14118=AXIS2_PLACEMENT_3D ( 'NONE', #25598, #18118, #27942 ) ;
#14139=DIRECTION ( 'NONE',  ( 0.000000000000000000, 0.000000000000000000, 1.000000000000000000 ) ) ;
#14153=CARTESIAN_POINT ( 'NONE',  ( -47.00000000000000000, 87.00000000000001421, 22.49999999999999289 ) ) ;
#14159=EDGE_LOOP ( 'NONE', ( #14007, #4647, #20299, #23670 ) ) ;
#14163=EDGE_CURVE ( 'NONE', #26039, #15359, #2695, .T. ) ;
#14173=ORIENTED_EDGE ( 'NONE', *, *, #10266, .F. ) ;
#14178=ORIENTED_EDGE ( 'NONE', *, *, #11303, .T. ) ;
#14181=DIRECTION ( 'NONE',  ( 0.000000000000000000, 0.000000000000000000, -1.000000000000000000 ) ) ;
#14187=AXIS2_PLACEMENT_3D ( 'NONE', #21708, #7385, #12207 ) ;
#14202=DIRECTION ( 'NONE',  ( -0.000000000000000000, 1.000000000000000000, -0.000000000000000000 ) ) ;
#14204=CARTESIAN_POINT ( 'NONE',  ( 4.510281037539698445E-13, -4.926614671774132148E-13, 77.49999999999998579 ) ) ;
#14208=CARTESIAN_POINT ( 'NONE',  ( -2.081668171172168513E-14, 75.00000000000001421, 37.49999999999999289 ) ) ;
#14215=DIRECTION ( 'NONE',  ( -0.000000000000000000, -0.000000000000000000, -1.000000000000000000 ) ) ;
#14219=DIRECTION ( 'NONE',  ( 0.000000000000000000, 0.000000000000000000, -1.000000000000000000 ) ) ;
#14231=CYLINDRICAL_SURFACE ( 'NONE', #24720, 3.000000000000002665 ) ;
#14245=CARTESIAN_POINT ( 'NONE',  ( 0.000000000000000000, 0.000000000000000000, 85.49999999999998579 ) ) ;
#14251=CARTESIAN_POINT ( 'NONE',  ( 37.99999999999999289, 65.00000000000000000, 50.49999999999998579 ) ) ;
#14266=TOROIDAL_SURFACE ( 'NONE', #15268, 53.00000000000000711, 3.000000000000000000 ) ;
#14281=CARTESIAN_POINT ( 'NONE',  ( -37.16608720827707657, -65.00000000000000000, 97.07879600563551037 ) ) ;
#14282=CARTESIAN_POINT ( 'NONE',  ( -70.00000000000000000, 65.00000000000000000, 12.49999999999999112 ) ) ;
#14306=CLOSED_SHELL ( 'NONE', ( #29193, #17137, #27110, #243, #19734, #30793, #9364, #5395, #17637, #1972, #26348, #12438, #30139, #12965, #14882, #5187, #22745, #12262, #12502, #6505, #4406, #2152, #19642, #5005, #23295, #2729, #3276, #2883, #15212, #10359, #234, #11525, #18307, #1947, #2992, #13433, #24889, #9216, #6518, #16154, #24603, #11464, #5556, #9003, #18699, #21420, #10930, #11340, #6329, #30509, #483, #27349, #14358, #18172, #12281, #7436, #19497, #14671, #26745, #20791, #6897, #27, #26522, #8793, #17134, #28823, #552, #15371, #1215, #16656, #21406, #29620, #422, #4431, #26951, #18004, #11678, #11829, #3300, #8629, #20234, #19507, #15297, #7000, #17964, #11542, #4247, #26765, #12615, #15514, #5181, #17749, #2563, #11895, #2138, #21394, #22314, #19704, #10134 ) ) ;
#14307=ORIENTED_EDGE ( 'NONE', *, *, #7718, .F. ) ;
#14340=ORIENTED_EDGE ( 'NONE', *, *, #16209, .T. ) ;
#14356=VECTOR ( 'NONE', #16980, 1000.000000000000000 ) ;
#14358=ADVANCED_FACE ( 'NONE', ( #6257 ), #22629, .F. ) ;
#14360=VERTEX_POINT ( 'NONE', #20456 ) ;
#14379=AXIS2_PLACEMENT_3D ( 'NONE', #14245, #7561, #14719 ) ;
#14393=CARTESIAN_POINT ( 'NONE',  ( 37.16608720827707657, -65.00000000000000000, 97.07879600563551037 ) ) ;
#14399=VERTEX_POINT ( 'NONE', #1729 ) ;
#14407=PRODUCT_DEFINITION_SHAPE ( 'NONE', 'NONE',  #24773 ) ;
#14422=EDGE_LOOP ( 'NONE', ( #14530, #2056, #27008, #25339 ) ) ;
#14463=DIRECTION ( 'NONE',  ( -1.000000000000000000, 0.000000000000000000, 0.000000000000000000 ) ) ;
#14496=EDGE_CURVE ( 'NONE', #1222, #27986, #21506, .T. ) ;
#14501=CARTESIAN_POINT ( 'NONE',  ( -37.16608720827707657, -51.86186943028246787, 97.07879600563551037 ) ) ;
#14508=EDGE_CURVE ( 'NONE', #5466, #27986, #12166, .T. ) ;
#14523=CARTESIAN_POINT ( 'NONE',  ( 49.67347041229598403, 69.99755012469657345, 55.05519839654500203 ) ) ;
#14530=ORIENTED_EDGE ( 'NONE', *, *, #23339, .T. ) ;
#14543=AXIS2_PLACEMENT_3D ( 'NONE', #21680, #21999, #12504 ) ;
#14558=DIRECTION ( 'NONE',  ( 0.000000000000000000, 0.000000000000000000, 1.000000000000000000 ) ) ;
#14564=CARTESIAN_POINT ( 'NONE',  ( 4.510281037539698445E-13, -4.926614671774132148E-13, 65.49999999999998579 ) ) ;
#14569=DIRECTION ( 'NONE',  ( -1.000000000000000000, 0.000000000000000000, 0.000000000000000000 ) ) ;
#14570=DIRECTION ( 'NONE',  ( -1.000000000000000000, 0.000000000000000000, 0.000000000000000000 ) ) ;
#14572=FACE_OUTER_BOUND ( 'NONE', #18465, .T. ) ;
#14583=DIRECTION ( 'NONE',  ( 0.000000000000000000, 0.000000000000000000, -1.000000000000000000 ) ) ;
#14585=ORIENTED_EDGE ( 'NONE', *, *, #12994, .T. ) ;
#14610=DIRECTION ( 'NONE',  ( -1.000000000000000000, 0.000000000000000000, 0.000000000000000000 ) ) ;
#14612=CARTESIAN_POINT ( 'NONE',  ( 4.510281037539698445E-13, -4.926614671774132148E-13, 82.49999999999998579 ) ) ;
#14613=CARTESIAN_POINT ( 'NONE',  ( -1.897971151300065476E-14, 75.00000000000001421, 22.49999999999999289 ) ) ;
#14629=VERTEX_POINT ( 'NONE', #29003 ) ;
#14633=ORIENTED_EDGE ( 'NONE', *, *, #4748, .T. ) ;
#14636=VECTOR ( 'NONE', #17267, 1000.000000000000000 ) ;
#14643=CARTESIAN_POINT ( 'NONE',  ( 4.510281037539698445E-13, -4.926614671774132148E-13, 82.49999999999998579 ) ) ;
#14650=ORIENTED_EDGE ( 'NONE', *, *, #1608, .T. ) ;
#14655=AXIS2_PLACEMENT_3D ( 'NONE', #17623, #19798, #14966 ) ;
#14670=CARTESIAN_POINT ( 'NONE',  ( 49.48768812108095005, 69.99365322046264737, 55.67629387500135607 ) ) ;
#14671=ADVANCED_FACE ( 'NONE', ( #1085 ), #10599, .T. ) ;
#14674=AXIS2_PLACEMENT_3D ( 'NONE', #3200, #9913, #24406 ) ;
#14681=DIRECTION ( 'NONE',  ( 0.000000000000000000, 0.000000000000000000, -1.000000000000000000 ) ) ;
#14693=CARTESIAN_POINT ( 'NONE',  ( -37.16608720827707657, -36.86186943028246787, 12.49999999999999112 ) ) ;
#14699=EDGE_CURVE ( 'NONE', #23537, #20897, #7657, .T. ) ;
#14712=EDGE_CURVE ( 'NONE', #30406, #20533, #6165, .T. ) ;
#14713=CARTESIAN_POINT ( 'NONE',  ( -50.00000000000000000, -50.00000000000000000, 62.49999999999999289 ) ) ;
#14719=DIRECTION ( 'NONE',  ( 1.000000000000000000, 0.000000000000000000, 0.000000000000000000 ) ) ;
#14734=CARTESIAN_POINT ( 'NONE',  ( -50.00000000000000000, 90.00000000000001421, 12.49999999999999112 ) ) ;
#14743=CARTESIAN_POINT ( 'NONE',  ( -70.00000000000000000, -70.00000000000000000, 12.49999999999999112 ) ) ;
#14767=CARTESIAN_POINT ( 'NONE',  ( -38.00000000000000000, 80.00000000000000000, -7.533656238527846826E-15 ) ) ;
#14772=AXIS2_PLACEMENT_3D ( 'NONE', #26552, #2375, #21397 ) ;
#14775=EDGE_LOOP ( 'NONE', ( #15277, #6924, #20671, #13369 ) ) ;
#14780=PLANE ( 'NONE',  #6997 ) ;
#14787=CIRCLE ( 'NONE', #18786, 17.00000000000000000 ) ;
#14788=DIRECTION ( 'NONE',  ( 1.000000000000000000, 0.000000000000000000, 0.000000000000000000 ) ) ;
#14797=VECTOR ( 'NONE', #640, 1000.000000000000000 ) ;
#14806=CARTESIAN_POINT ( 'NONE',  ( 37.99999999999933920, 0.000000000000000000, 85.49999999999998579 ) ) ;
#14819=EDGE_LOOP ( 'NONE', ( #15727, #23341, #9340, #25609 ) ) ;
#14820=AXIS2_PLACEMENT_3D ( 'NONE', #30650, #19273, #18824 ) ;
#14831=CIRCLE ( 'NONE', #24813, 5.000000000000004441 ) ;
#14836=DIRECTION ( 'NONE',  ( 0.000000000000000000, 1.000000000000000000, 0.000000000000000000 ) ) ;
#14860=VERTEX_POINT ( 'NONE', #8720 ) ;
#14864=CARTESIAN_POINT ( 'NONE',  ( 0.000000000000000000, 65.00000000000000000, 50.49999999999998579 ) ) ;
#14866=AXIS2_PLACEMENT_3D ( 'NONE', #19404, #28463, #2243 ) ;
#14876=ORIENTED_EDGE ( 'NONE', *, *, #14117, .T. ) ;
#14878=FACE_OUTER_BOUND ( 'NONE', #7559, .T. ) ;
#14882=ADVANCED_FACE ( 'NONE', ( #1244 ), #6068, .F. ) ;
#14887=EDGE_LOOP ( 'NONE', ( #9878, #26987, #18795, #4009, #2780, #18507, #21138, #1861, #16577, #1118 ) ) ;
#14888=CARTESIAN_POINT ( 'NONE',  ( -70.00000000000000000, 50.00000000000000000, 59.49999999999999289 ) ) ;
#14889=CARTESIAN_POINT ( 'NONE',  ( -40.00000000000002842, 80.00000000000001421, 57.50000000000015632 ) ) ;
#14892=CARTESIAN_POINT ( 'NONE',  ( -50.00000000000000000, 50.00000000000000000, 62.49999999999999289 ) ) ;
#14895=LINE ( 'NONE', #3048, #5955 ) ;
#14903=EDGE_CURVE ( 'NONE', #10854, #22904, #13141, .T. ) ;
#14914=DIRECTION ( 'NONE',  ( 0.000000000000000000, 0.000000000000000000, -1.000000000000000000 ) ) ;
#14917=LINE ( 'NONE', #17567, #9789 ) ;
#14923=EDGE_CURVE ( 'NONE', #19418, #24377, #18745, .T. ) ;
#14924=FACE_OUTER_BOUND ( 'NONE', #13475, .T. ) ;
#14925=VECTOR ( 'NONE', #21879, 1000.000000000000000 ) ;
#14940=CARTESIAN_POINT ( 'NONE',  ( 0.000000000000000000, 90.00000000000001421, 0.000000000000000000 ) ) ;
#14960=EDGE_LOOP ( 'NONE', ( #11462, #7152, #17294, #22608 ) ) ;
#14966=DIRECTION ( 'NONE',  ( 0.000000000000000000, 0.000000000000000000, 1.000000000000000000 ) ) ;
#14982=CARTESIAN_POINT ( 'NONE',  ( 37.16608720827707657, 36.86186943028246787, 97.07879600563551037 ) ) ;
#14985=EDGE_CURVE ( 'NONE', #10252, #10893, #12453, .T. ) ;
#14995=LINE ( 'NONE', #24827, #8761 ) ;
#15007=ORIENTED_EDGE ( 'NONE', *, *, #10197, .T. ) ;
#15013=DIRECTION ( 'NONE',  ( 1.982541115402065110E-16, 0.000000000000000000, -1.000000000000000000 ) ) ;
#15058=VECTOR ( 'NONE', #30837, 1000.000000000000000 ) ;
#15059=CARTESIAN_POINT ( 'NONE',  ( -49.73013633871049421, 69.99829191145150276, 20.16832805650060934 ) ) ;
#15085=EDGE_CURVE ( 'NONE', #22374, #346, #7605, .T. ) ;
#15098=VECTOR ( 'NONE', #26361, 1000.000000000000000 ) ;
#15100=LINE ( 'NONE', #5287, #14356 ) ;
#15108=VERTEX_POINT ( 'NONE', #19454 ) ;
#15114=LINE ( 'NONE', #3264, #2208 ) ;
#15118=AXIS2_PLACEMENT_3D ( 'NONE', #9121, #4281, #20405 ) ;
#15133=CARTESIAN_POINT ( 'NONE',  ( -37.16608720827707657, 36.86186943028246787, 97.07879600563551037 ) ) ;
#15136=CARTESIAN_POINT ( 'NONE',  ( -57.50000000000001421, 50.00000000000000000, 97.07879600563551037 ) ) ;
#15137=DIRECTION ( 'NONE',  ( 0.000000000000000000, -1.000000000000000000, 0.000000000000000000 ) ) ;
#15140=CARTESIAN_POINT ( 'NONE',  ( -4.163336342344337027E-14, 1.387778780781445676E-14, 77.49999999999998579 ) ) ;
#15155=ORIENTED_EDGE ( 'NONE', *, *, #10180, .T. ) ;
#15167=LINE ( 'NONE', #19552, #21288 ) ;
#15174=FACE_OUTER_BOUND ( 'NONE', #18882, .T. ) ;
#15177=DIRECTION ( 'NONE',  ( 0.000000000000000000, 0.000000000000000000, 1.000000000000000000 ) ) ;
#15180=VERTEX_POINT ( 'NONE', #11026 ) ;
#15193=ORIENTED_EDGE ( 'NONE', *, *, #20200, .F. ) ;
#15202=DIRECTION ( 'NONE',  ( 0.000000000000000000, 0.000000000000000000, -1.000000000000000000 ) ) ;
#15208=CARTESIAN_POINT ( 'NONE',  ( -38.00000000000000000, 80.00000000000000000, -7.533656238527846826E-15 ) ) ;
#15212=ADVANCED_FACE ( 'NONE', ( #8835 ), #10871, .T. ) ;
#15213=PLANE ( 'NONE',  #21918 ) ;
#15219=ORIENTED_EDGE ( 'NONE', *, *, #20349, .T. ) ;
#15230=ORIENTED_EDGE ( 'NONE', *, *, #20682, .F. ) ;
#15236=CARTESIAN_POINT ( 'NONE',  ( 37.99999999999999289, 80.00000000000000000, 0.000000000000000000 ) ) ;
#15249=ORIENTED_EDGE ( 'NONE', *, *, #6115, .F. ) ;
#15253=EDGE_CURVE ( 'NONE', #9249, #23905, #29241, .T. ) ;
#15262=EDGE_CURVE ( 'NONE', #19317, #5791, #11657, .T. ) ;
#15264=VECTOR ( 'NONE', #17119, 1000.000000000000000 ) ;
#15268=AXIS2_PLACEMENT_3D ( 'NONE', #14564, #671, #24060 ) ;
#15277=ORIENTED_EDGE ( 'NONE', *, *, #6448, .T. ) ;
#15281=DIRECTION ( 'NONE',  ( 0.000000000000000000, 0.000000000000000000, 1.000000000000000000 ) ) ;
#15282=FACE_OUTER_BOUND ( 'NONE', #3015, .T. ) ;
#15289=CARTESIAN_POINT ( 'NONE',  ( 37.99999999999999289, 80.00000000000001421, 47.91742430504415040 ) ) ;
#15292=CARTESIAN_POINT ( 'NONE',  ( 43.65325317339704014, 67.82531247263540308, 61.81444804503984614 ) ) ;
#15297=ADVANCED_FACE ( 'NONE', ( #2738 ), #4174, .T. ) ;
#15307=EDGE_CURVE ( 'NONE', #24053, #10610, #27097, .T. ) ;
#15308=CIRCLE ( 'NONE', #16810, 4.999999999999997335 ) ;
#15313=VERTEX_POINT ( 'NONE', #26087 ) ;
#15337=DIRECTION ( 'NONE',  ( 0.000000000000000000, 0.000000000000000000, -1.000000000000000000 ) ) ;
#15344=AXIS2_PLACEMENT_3D ( 'NONE', #5053, #11758, #30784 ) ;
#15359=VERTEX_POINT ( 'NONE', #18932 ) ;
#15361=DIRECTION ( 'NONE',  ( 0.000000000000000000, 1.000000000000000000, 0.000000000000000000 ) ) ;
#15362=VECTOR ( 'NONE', #21636, 1000.000000000000000 ) ;
#15371=ADVANCED_FACE ( 'NONE', ( #30459 ), #9102, .T. ) ;
#15373=DIRECTION ( 'NONE',  ( 0.000000000000000000, 0.000000000000000000, 1.000000000000000000 ) ) ;
#15376=CARTESIAN_POINT ( 'NONE',  ( 0.000000000000000000, 87.00000000000001421, 15.49999999999998934 ) ) ;
#15394=CARTESIAN_POINT ( 'NONE',  ( -47.00000000000000000, 90.00000000000001421, 22.49999999999999289 ) ) ;
#15399=CIRCLE ( 'NONE', #29356, 47.00000000000000000 ) ;
#15405=VECTOR ( 'NONE', #22293, 1000.000000000000000 ) ;
#15418=CARTESIAN_POINT ( 'NONE',  ( 48.92864595558773999, 69.97303745521041662, 17.94690505038828121 ) ) ;
#15427=CIRCLE ( 'NONE', #16412, 3.000000000000002665 ) ;
#15443=CARTESIAN_POINT ( 'NONE',  ( 49.99999999999998579, -70.00000000000000000, 12.49999999999999112 ) ) ;
#15454=CARTESIAN_POINT ( 'NONE',  ( 42.73635331409263927, 67.00059091328013494, 62.14018542721996141 ) ) ;
#15455=ORIENTED_EDGE ( 'NONE', *, *, #9602, .T. ) ;
#15457=CARTESIAN_POINT ( 'NONE',  ( -43.96625599154361197, 68.08820126035209341, 61.68658881044186870 ) ) ;
#15465=LINE ( 'NONE', #29518, #16390 ) ;
#15466=ORIENTED_EDGE ( 'NONE', *, *, #8811, .T. ) ;
#15470=LINE ( 'NONE', #27496, #19939 ) ;
#15477=DIRECTION ( 'NONE',  ( -0.000000000000000000, -0.000000000000000000, 1.000000000000000000 ) ) ;
#15485=EDGE_CURVE ( 'NONE', #29733, #886, #12793, .T. ) ;
#15500=ORIENTED_EDGE ( 'NONE', *, *, #20200, .T. ) ;
#15502=CARTESIAN_POINT ( 'NONE',  ( 0.000000000000000000, 90.00000000000001421, 15.49999999999998934 ) ) ;
#15509=EDGE_CURVE ( 'NONE', #3904, #12729, #10679, .T. ) ;
#15514=ADVANCED_FACE ( 'NONE', ( #12491 ), #24790, .T. ) ;
#15521=LINE ( 'NONE', #13194, #21805 ) ;
#15523=EDGE_LOOP ( 'NONE', ( #9512, #26001, #25762, #5093 ) ) ;
#15528=CARTESIAN_POINT ( 'NONE',  ( -50.00000000000000000, 70.00000000000000000, 22.49999999999999289 ) ) ;
#15531=LINE ( 'NONE', #11170, #28442 ) ;
#15536=DIRECTION ( 'NONE',  ( 0.000000000000000000, 0.000000000000000000, 1.000000000000000000 ) ) ;
#15551=DIRECTION ( 'NONE',  ( 1.000000000000000000, 0.000000000000000000, 0.000000000000000000 ) ) ;
#15561=CARTESIAN_POINT ( 'NONE',  ( -40.00000000000000000, -0.000000000000000000, 62.49999999999999289 ) ) ;
#15564=CARTESIAN_POINT ( 'NONE',  ( 37.16608720827707657, -51.86186943028246787, 97.07879600563551037 ) ) ;
#15573=ORIENTED_EDGE ( 'NONE', *, *, #25413, .T. ) ;
#15575=CARTESIAN_POINT ( 'NONE',  ( 47.81953956977370979, 69.88199567761851938, 16.25762515829667976 ) ) ;
#15578=DIRECTION ( 'NONE',  ( -0.000000000000000000, -0.000000000000000000, -1.000000000000000000 ) ) ;
#15584=FACE_OUTER_BOUND ( 'NONE', #7940, .T. ) ;
#15598=DIRECTION ( 'NONE',  ( 0.000000000000000000, 1.000000000000000000, 0.000000000000000000 ) ) ;
#15599=CARTESIAN_POINT ( 'NONE',  ( -38.00000000000000711, 80.00000000000001421, 50.49999999999998579 ) ) ;
#15619=AXIS2_PLACEMENT_3D ( 'NONE', #19632, #21980, #26666 ) ;
#15627=VERTEX_POINT ( 'NONE', #761 ) ;
#15638=EDGE_CURVE ( 'NONE', #9325, #12261, #15114, .T. ) ;
#15639=AXIS2_PLACEMENT_3D ( 'NONE', #10209, #23938, #24239 ) ;
#15643=ORIENTED_EDGE ( 'NONE', *, *, #28270, .T. ) ;
#15648=CARTESIAN_POINT ( 'NONE',  ( 49.99999999999998579, -50.00000000000000000, 12.49999999999999112 ) ) ;
#15664=CARTESIAN_POINT ( 'NONE',  ( -52.16608720827707657, 51.86186943028246787, 57.49999999999999289 ) ) ;
#15691=DIRECTION ( 'NONE',  ( 0.000000000000000000, 0.000000000000000000, -1.000000000000000000 ) ) ;
#15716=CIRCLE ( 'NONE', #30713, 5.000000000000004441 ) ;
#15726=EDGE_LOOP ( 'NONE', ( #4335, #19932, #24501, #11211, #22872, #1133 ) ) ;
#15727=ORIENTED_EDGE ( 'NONE', *, *, #10922, .T. ) ;
#15733=CARTESIAN_POINT ( 'NONE',  ( -40.00000000000000000, 87.00000000000001421, 12.49999999999999112 ) ) ;
#15743=EDGE_LOOP ( 'NONE', ( #5215, #24365, #7335, #7193, #26723, #16037 ) ) ;
#15745=PRODUCT_DEFINITION_CONTEXT ( 'detailed design', #25330, 'design' ) ;
#15750=AXIS2_PLACEMENT_3D ( 'NONE', #8635, #8328, #11271 ) ;
#15752=DIRECTION ( 'NONE',  ( 0.000000000000000000, 0.000000000000000000, 1.000000000000000000 ) ) ;
#15781=DIRECTION ( 'NONE',  ( 0.000000000000000000, 0.000000000000000000, 1.000000000000000000 ) ) ;
#15782=ORIENTED_EDGE ( 'NONE', *, *, #4748, .F. ) ;
#15798=VERTEX_POINT ( 'NONE', #16505 ) ;
#15831=AXIS2_PLACEMENT_3D ( 'NONE', #28001, #28470, #7095 ) ;
#15842=PLANE ( 'NONE',  #18823 ) ;
#15851=CARTESIAN_POINT ( 'NONE',  ( 4.510281037539698445E-13, -4.926614671774132148E-13, 65.49999999999998579 ) ) ;
#15861=CARTESIAN_POINT ( 'NONE',  ( 39.99999999999998579, 87.00000000000001421, 62.49999999999999289 ) ) ;
#15862=EDGE_CURVE ( 'NONE', #24493, #24670, #1705, .T. ) ;
#15863=ORIENTED_EDGE ( 'NONE', *, *, #381, .F. ) ;
#15864=ORIENTED_EDGE ( 'NONE', *, *, #12056, .F. ) ;
#15884=CIRCLE ( 'NONE', #14379, 34.99999999999933920 ) ;
#15904=AXIS2_PLACEMENT_3D ( 'NONE', #3972, #20492, #8654 ) ;
#15921=VERTEX_POINT ( 'NONE', #5887 ) ;
#15935=ORIENTED_EDGE ( 'NONE', *, *, #30731, .F. ) ;
#15944=VERTEX_POINT ( 'NONE', #24126 ) ;
#15957=DIRECTION ( 'NONE',  ( 0.000000000000000000, 1.000000000000000000, 0.000000000000000000 ) ) ;
#15969=DIRECTION ( 'NONE',  ( 0.000000000000000000, 0.000000000000000000, -1.000000000000000000 ) ) ;
#15984=VERTEX_POINT ( 'NONE', #23167 ) ;
#15994=CARTESIAN_POINT ( 'NONE',  ( -44.79023165781732274, 69.31820106020313688, 13.69674458689816454 ) ) ;
#16008=ORIENTED_EDGE ( 'NONE', *, *, #2498, .F. ) ;
#16012=EDGE_CURVE ( 'NONE', #22374, #9580, #3722, .T. ) ;
#16020=PLANE ( 'NONE',  #25307 ) ;
#16029=CARTESIAN_POINT ( 'NONE',  ( -50.00000000000000000, 50.00000000000000000, 62.49999999999999289 ) ) ;
#16037=ORIENTED_EDGE ( 'NONE', *, *, #23833, .F. ) ;
#16038=B_SPLINE_CURVE_WITH_KNOTS ( 'NONE', 3,
 ( #10164, #17181, #29512, #24356, #17502, #7683, #19671, #29662, #3299, #15457, #3003, #12982, #7832, #1120, #22472, #29360 ),
 .UNSPECIFIED., .F., .F.,
 ( 4, 2, 2, 2, 2, 2, 2, 4 ),
 ( 3.030954607830198967E-16, 0.001284364552519681778, 0.001926546828779363832, 0.002568729105039046102, 0.003853093657558390259, 0.005137458210077733983, 0.007706187315116445717, 0.01027491642015515745 ),
 .UNSPECIFIED. ) ;
#16042=EDGE_LOOP ( 'NONE', ( #2694, #20038, #93, #12241 ) ) ;
#16046=VERTEX_POINT ( 'NONE', #15861 ) ;
#16053=EDGE_CURVE ( 'NONE', #4577, #28559, #27716, .T. ) ;
#16069=AXIS2_PLACEMENT_3D ( 'NONE', #15133, #29028, #3284 ) ;
#16079=VERTEX_POINT ( 'NONE', #16320 ) ;
#16095=FACE_OUTER_BOUND ( 'NONE', #25093, .T. ) ;
#16097=EDGE_CURVE ( 'NONE', #12285, #15984, #19725, .T. ) ;
#16104=DIRECTION ( 'NONE',  ( 0.000000000000000000, 1.000000000000000000, 0.000000000000000000 ) ) ;
#16117=EDGE_CURVE ( 'NONE', #4652, #19850, #29248, .T. ) ;
#16135=ORIENTED_EDGE ( 'NONE', *, *, #16605, .F. ) ;
#16140=CARTESIAN_POINT ( 'NONE',  ( -40.00000000000002842, 80.00000000000001421, 22.49999999999983302 ) ) ;
#16144=PLANE ( 'NONE',  #23691 ) ;
#16154=ADVANCED_FACE ( 'NONE', ( #2744 ), #7736, .F. ) ;
#16157=LINE ( 'NONE', #23468, #20908 ) ;
#16172=CARTESIAN_POINT ( 'NONE',  ( 52.16608720827707657, -51.86186943028246787, 97.07879600563551037 ) ) ;
#16209=EDGE_CURVE ( 'NONE', #30732, #2852, #5711, .T. ) ;
#16214=ORIENTED_EDGE ( 'NONE', *, *, #26901, .F. ) ;
#16230=EDGE_CURVE ( 'NONE', #27312, #10762, #1019, .T. ) ;
#16243=ORIENTED_EDGE ( 'NONE', *, *, #201, .F. ) ;
#16277=AXIS2_PLACEMENT_3D ( 'NONE', #3034, #2727, #12234 ) ;
#16288=VECTOR ( 'NONE', #26225, 1000.000000000000000 ) ;
#16318=VECTOR ( 'NONE', #8109, 1000.000000000000000 ) ;
#16320=CARTESIAN_POINT ( 'NONE',  ( 37.16608720827707657, 65.00000000000000000, 12.49999999999999112 ) ) ;
#16321=AXIS2_PLACEMENT_3D ( 'NONE', #19729, #22389, #28949 ) ;
#16340=CARTESIAN_POINT ( 'NONE',  ( -57.50000000000001421, -50.00000000000000000, 62.49999999999999289 ) ) ;
#16341=DIRECTION ( 'NONE',  ( 0.000000000000000000, 0.000000000000000000, -1.000000000000000000 ) ) ;
#16353=CARTESIAN_POINT ( 'NONE',  ( -49.01087064057495724, 69.97702420031504289, 56.88420116493780654 ) ) ;
#16354=CYLINDRICAL_SURFACE ( 'NONE', #13857, 7.500000000000000000 ) ;
#16379=EDGE_LOOP ( 'NONE', ( #17409, #30133, #817, #3932, #28049, #7401 ) ) ;
#16382=CARTESIAN_POINT ( 'NONE',  ( 64.99999999999998579, 36.86186943028246787, 57.49999999999999289 ) ) ;
#16390=VECTOR ( 'NONE', #22177, 1000.000000000000000 ) ;
#16410=ORIENTED_EDGE ( 'NONE', *, *, #1327, .T. ) ;
#16412=AXIS2_PLACEMENT_3D ( 'NONE', #19155, #21017, #26169 ) ;
#16423=CARTESIAN_POINT ( 'NONE',  ( 37.16608720827707657, 65.00000000000000000, 97.07879600563551037 ) ) ;
#16444=DIRECTION ( 'NONE',  ( 0.000000000000000000, -1.000000000000000000, 0.000000000000000000 ) ) ;
#16456=CARTESIAN_POINT ( 'NONE',  ( 69.99999999999998579, 50.00000000000000000, 59.49999999999999289 ) ) ;
#16458=LINE ( 'NONE', #8987, #963 ) ;
#16461=DIRECTION ( 'NONE',  ( 0.000000000000000000, 0.000000000000000000, 1.000000000000000000 ) ) ;
#16462=VERTEX_POINT ( 'NONE', #19389 ) ;
#16463=ORIENTED_EDGE ( 'NONE', *, *, #4260, .F. ) ;
#16498=ORIENTED_EDGE ( 'NONE', *, *, #22144, .T. ) ;
#16499=ORIENTED_EDGE ( 'NONE', *, *, #207, .T. ) ;
#16505=CARTESIAN_POINT ( 'NONE',  ( -1.897971151300065476E-14, 80.00000000000000000, 22.49999999999999289 ) ) ;
#16509=CARTESIAN_POINT ( 'NONE',  ( -50.00000000000000000, 70.00000000000000000, 52.49999999999999289 ) ) ;
#16529=FACE_OUTER_BOUND ( 'NONE', #26100, .T. ) ;
#16560=ORIENTED_EDGE ( 'NONE', *, *, #15638, .T. ) ;
#16566=VERTEX_POINT ( 'NONE', #24673 ) ;
#16576=DIRECTION ( 'NONE',  ( 1.000000000000000000, 0.000000000000000000, 0.000000000000000000 ) ) ;
#16577=ORIENTED_EDGE ( 'NONE', *, *, #21570, .F. ) ;
#16584=ORIENTED_EDGE ( 'NONE', *, *, #6530, .T. ) ;
#16585=ORIENTED_EDGE ( 'NONE', *, *, #12452, .F. ) ;
#16591=ORIENTED_EDGE ( 'NONE', *, *, #9602, .F. ) ;
#16594=CYLINDRICAL_SURFACE ( 'NONE', #14866, 4.999999999999997335 ) ;
#16605=EDGE_CURVE ( 'NONE', #10893, #4652, #3313, .T. ) ;
#16620=AXIS2_PLACEMENT_3D ( 'NONE', #28072, #28214, #6697 ) ;
#16655=ORIENTED_EDGE ( 'NONE', *, *, #3282, .T. ) ;
#16656=ADVANCED_FACE ( 'NONE', ( #18896 ), #13749, .F. ) ;
#16660=DIRECTION ( 'NONE',  ( 0.000000000000000000, -0.000000000000000000, 1.000000000000000000 ) ) ;
#16662=EDGE_CURVE ( 'NONE', #25790, #8546, #8738, .T. ) ;
#16695=ORIENTED_EDGE ( 'NONE', *, *, #28061, .T. ) ;
#16703=UNCERTAINTY_MEASURE_WITH_UNIT (LENGTH_MEASURE( 1.000000000000000082E-05 ), #9309, 'distance_accuracy_value', 'NONE');
#16712=DIRECTION ( 'NONE',  ( -0.000000000000000000, -0.000000000000000000, -1.000000000000000000 ) ) ;
#16715=CARTESIAN_POINT ( 'NONE',  ( 69.99999999999998579, -50.00000000000000000, 12.49999999999999112 ) ) ;
#16729=ORIENTED_EDGE ( 'NONE', *, *, #29199, .T. ) ;
#16738=ORIENTED_EDGE ( 'NONE', *, *, #6742, .F. ) ;
#16747=CARTESIAN_POINT ( 'NONE',  ( -2.081668171172168513E-14, 75.00000000000001421, 37.49999999999999289 ) ) ;
#16751=CYLINDRICAL_SURFACE ( 'NONE', #1868, 15.00000000000000000 ) ;
#16763=AXIS2_PLACEMENT_3D ( 'NONE', #20305, #29832, #8303 ) ;
#16772=VECTOR ( 'NONE', #27240, 1000.000000000000000 ) ;
#16775=CARTESIAN_POINT ( 'NONE',  ( 39.99999999999998579, 80.00000000000001421, 52.49999999999999289 ) ) ;
#16788=EDGE_CURVE ( 'NONE', #346, #29075, #29155, .T. ) ;
#16790=CARTESIAN_POINT ( 'NONE',  ( 64.99999999999998579, 36.86186943028246787, 97.07879600563551037 ) ) ;
#16803=EDGE_CURVE ( 'NONE', #14860, #15627, #21838, .T. ) ;
#16807=CARTESIAN_POINT ( 'NONE',  ( -49.75043292984307897, 69.99853936330177362, 54.74343500730861223 ) ) ;
#16808=CIRCLE ( 'NONE', #23759, 5.000000000000004441 ) ;
#16810=AXIS2_PLACEMENT_3D ( 'NONE', #8740, #18260, #8906 ) ;
#16839=EDGE_CURVE ( 'NONE', #14360, #25524, #24483, .T. ) ;
#16884=CARTESIAN_POINT ( 'NONE',  ( 4.510281037539698445E-13, -4.926614671774132148E-13, 79.49999999999998579 ) ) ;
#16885=CYLINDRICAL_SURFACE ( 'NONE', #10285, 4.999999999999997335 ) ;
#16903=TOROIDAL_SURFACE ( 'NONE', #1468, 37.99999999999933920, 3.000000000000000000 ) ;
#16920=LINE ( 'NONE', #28773, #3459 ) ;
#16924=ORIENTED_EDGE ( 'NONE', *, *, #22910, .F. ) ;
#16945=CARTESIAN_POINT ( 'NONE',  ( 37.16608720827707657, 65.00000000000000000, 57.49999999999999289 ) ) ;
#16954=CARTESIAN_POINT ( 'NONE',  ( -46.99999999999955236, -4.869056272214205871E-13, 79.49999999999998579 ) ) ;
#16969=CARTESIAN_POINT ( 'NONE',  ( 49.99999999999998579, -50.00000000000000000, 62.49999999999999289 ) ) ;
#16975=CARTESIAN_POINT ( 'NONE',  ( -2.081668171172168513E-14, 80.00000000000000000, 37.49999999999999289 ) ) ;
#16980=DIRECTION ( 'NONE',  ( -0.000000000000000000, -1.000000000000000000, 0.000000000000000000 ) ) ;
#16994=EDGE_CURVE ( 'NONE', #13279, #30435, #30654, .T. ) ;
#17000=DIRECTION ( 'NONE',  ( 0.000000000000000000, 0.000000000000000000, -1.000000000000000000 ) ) ;
#17038=DIRECTION ( 'NONE',  ( -0.000000000000000000, -0.000000000000000000, 1.000000000000000000 ) ) ;
#17064=DIRECTION ( 'NONE',  ( -0.000000000000000000, -1.000000000000000000, -0.000000000000000000 ) ) ;
#17069=CARTESIAN_POINT ( 'NONE',  ( -70.00000000000000000, -70.00000000000000000, 12.49999999999999112 ) ) ;
#17076=CARTESIAN_POINT ( 'NONE',  ( 49.99999999999998579, 50.00000000000000000, 59.49999999999999289 ) ) ;
#17079=ORIENTED_EDGE ( 'NONE', *, *, #13466, .T. ) ;
#17090=CIRCLE ( 'NONE', #23551, 2.999999999999999112 ) ;
#17102=CARTESIAN_POINT ( 'NONE',  ( 14.99999999999995737, 1.387778780781445676E-14, 67.49999999999997158 ) ) ;
#17107=AXIS2_PLACEMENT_3D ( 'NONE', #2570, #6941, #7405 ) ;
#17119=DIRECTION ( 'NONE',  ( -0.000000000000000000, -0.000000000000000000, 1.000000000000000000 ) ) ;
#17122=ORIENTED_EDGE ( 'NONE', *, *, #17188, .T. ) ;
#17124=ORIENTED_EDGE ( 'NONE', *, *, #20679, .T. ) ;
#17128=CARTESIAN_POINT ( 'NONE',  ( 37.16608720827707657, -36.86186943028246787, 12.49999999999999112 ) ) ;
#17134=ADVANCED_FACE ( 'NONE', ( #7898 ), #26925, .T. ) ;
#17135=DIRECTION ( 'NONE',  ( -0.000000000000000000, 1.000000000000000000, 0.000000000000000000 ) ) ;
#17137=ADVANCED_FACE ( 'NONE', ( #702 ), #19429, .F. ) ;
#17143=CARTESIAN_POINT ( 'NONE',  ( -38.00000000000000711, 80.00000000000000000, 50.49999999999998579 ) ) ;
#17155=CARTESIAN_POINT ( 'NONE',  ( 49.99999999999998579, 87.00000000000001421, 52.49999999999999289 ) ) ;
#17181=CARTESIAN_POINT ( 'NONE',  ( -46.83962922035959053, 69.75107690209843270, 59.80789677786150094 ) ) ;
#17188=EDGE_CURVE ( 'NONE', #20591, #29733, #6754, .T. ) ;
#17198=DIRECTION ( 'NONE',  ( 0.000000000000000000, 1.000000000000000000, 0.000000000000000000 ) ) ;
#17215=EDGE_LOOP ( 'NONE', ( #4612, #24754, #6191, #29495, #569, #3399, #2767, #29690, #15007, #26945 ) ) ;
#17225=DIRECTION ( 'NONE',  ( -0.000000000000000000, -0.000000000000000000, 1.000000000000000000 ) ) ;
#17235=CIRCLE ( 'NONE', #1301, 10.00000000000000178 ) ;
#17247=VECTOR ( 'NONE', #2834, 1000.000000000000000 ) ;
#17266=AXIS2_PLACEMENT_3D ( 'NONE', #28112, #16104, #23257 ) ;
#17267=DIRECTION ( 'NONE',  ( -0.000000000000000000, -0.000000000000000000, -1.000000000000000000 ) ) ;
#17269=AXIS2_PLACEMENT_3D ( 'NONE', #3688, #712, #13052 ) ;
#17276=CARTESIAN_POINT ( 'NONE',  ( 64.99999999999998579, -70.00000000000000000, 12.49999999999999112 ) ) ;
#17294=ORIENTED_EDGE ( 'NONE', *, *, #13785, .F. ) ;
#17304=CIRCLE ( 'NONE', #21775, 10.00000000000000178 ) ;
#17312=VECTOR ( 'NONE', #29383, 1000.000000000000000 ) ;
#17326=CARTESIAN_POINT ( 'NONE',  ( 49.93671616582084738, 70.00028419060272711, 53.79459073512090583 ) ) ;
#17330=VECTOR ( 'NONE', #21300, 1000.000000000000000 ) ;
#17336=CARTESIAN_POINT ( 'NONE',  ( -34.99999999999933920, 0.000000000000000000, 85.49999999999998579 ) ) ;
#17341=CIRCLE ( 'NONE', #29804, 15.00000000000000000 ) ;
#17342=LINE ( 'NONE', #26871, #21682 ) ;
#17359=ORIENTED_EDGE ( 'NONE', *, *, #21962, .T. ) ;
#17361=EDGE_CURVE ( 'NONE', #16046, #4862, #21546, .T. ) ;
#17376=CARTESIAN_POINT ( 'NONE',  ( -52.16608720827707657, -36.86186943028246787, 57.49999999999999289 ) ) ;
#17379=ORIENTED_EDGE ( 'NONE', *, *, #15262, .T. ) ;
#17380=AXIS2_PLACEMENT_3D ( 'NONE', #17434, #7606, #9949 ) ;
#17388=ORIENTED_EDGE ( 'NONE', *, *, #3298, .T. ) ;
#17397=EDGE_CURVE ( 'NONE', #19418, #27728, #16038, .T. ) ;
#17404=EDGE_CURVE ( 'NONE', #8240, #23407, #14995, .T. ) ;
#17409=ORIENTED_EDGE ( 'NONE', *, *, #7863, .F. ) ;
#17425=VERTEX_POINT ( 'NONE', #29192 ) ;
#17427=DIRECTION ( 'NONE',  ( -0.000000000000000000, -1.000000000000000000, -0.000000000000000000 ) ) ;
#17431=VERTEX_POINT ( 'NONE', #648 ) ;
#17432=CARTESIAN_POINT ( 'NONE',  ( -50.00000000000000000, -70.00000000000000000, 12.49999999999999112 ) ) ;
#17433=EDGE_CURVE ( 'NONE', #20557, #26276, #17342, .T. ) ;
#17434=CARTESIAN_POINT ( 'NONE',  ( -2.081668171172168513E-14, 90.00000000000001421, 37.49999999999999289 ) ) ;
#17449=ORIENTED_EDGE ( 'NONE', *, *, #2683, .T. ) ;
#17453=DIRECTION ( 'NONE',  ( -1.000000000000000000, 0.000000000000000000, 0.000000000000000000 ) ) ;
#17462=CARTESIAN_POINT ( 'NONE',  ( 39.99999999999998579, 80.00000000000001421, 22.49999999999999289 ) ) ;
#17480=CARTESIAN_POINT ( 'NONE',  ( 49.99999999999998579, -67.00000000000000000, 62.49999999999999289 ) ) ;
#17502=CARTESIAN_POINT ( 'NONE',  ( -45.88720696345781391, 69.36824176953101073, 60.58574796622433212 ) ) ;
#17504=CARTESIAN_POINT ( 'NONE',  ( 0.000000000000000000, 0.000000000000000000, 92.49999999999998579 ) ) ;
#17521=DIRECTION ( 'NONE',  ( 0.000000000000000000, 0.000000000000000000, 1.000000000000000000 ) ) ;
#17536=EDGE_CURVE ( 'NONE', #509, #977, #7525, .T. ) ;
#17545=VECTOR ( 'NONE', #3253, 1000.000000000000000 ) ;
#17548=DIRECTION ( 'NONE',  ( -1.000000000000000000, 0.000000000000000000, 0.000000000000000000 ) ) ;
#17549=EDGE_CURVE ( 'NONE', #11497, #20113, #7780, .T. ) ;
#17558=CARTESIAN_POINT ( 'NONE',  ( 0.000000000000000000, 0.000000000000000000, 62.49999999999999289 ) ) ;
#17562=VECTOR ( 'NONE', #24243, 1000.000000000000000 ) ;
#17567=CARTESIAN_POINT ( 'NONE',  ( -7.483314773547907528, 75.00000000000001421, 50.49999999999998579 ) ) ;
#17579=CARTESIAN_POINT ( 'NONE',  ( 37.99999999999999289, 80.00000000000000000, 0.000000000000000000 ) ) ;
#17597=EDGE_CURVE ( 'NONE', #17807, #22741, #30205, .T. ) ;
#17602=DIRECTION ( 'NONE',  ( -0.000000000000000000, -0.000000000000000000, -1.000000000000000000 ) ) ;
#17623=CARTESIAN_POINT ( 'NONE',  ( -40.00000000000000000, 90.00000000000001421, 52.49999999999999289 ) ) ;
#17637=ADVANCED_FACE ( 'NONE', ( #28080 ), #20893, .F. ) ;
#17642=DIRECTION ( 'NONE',  ( 0.000000000000000000, 0.000000000000000000, -1.000000000000000000 ) ) ;
#17644=LINE ( 'NONE', #15136, #30324 ) ;
#17683=CARTESIAN_POINT ( 'NONE',  ( -70.00000000000000000, -70.00000000000000000, 12.49999999999999112 ) ) ;
#17691=LINE ( 'NONE', #15502, #8937 ) ;
#17717=DIRECTION ( 'NONE',  ( -1.000000000000000000, 0.000000000000000000, 0.000000000000000000 ) ) ;
#17729=AXIS2_PLACEMENT_3D ( 'NONE', #16954, #24579, #719 ) ;
#17736=CIRCLE ( 'NONE', #2783, 7.500000000000000000 ) ;
#17749=ADVANCED_FACE ( 'NONE', ( #7956 ), #19484, .T. ) ;
#17777=LINE ( 'NONE', #19800, #15405 ) ;
#17790=EDGE_LOOP ( 'NONE', ( #27464, #25950 ) ) ;
#17792=AXIS2_PLACEMENT_3D ( 'NONE', #14208, #11896, #31 ) ;
#17794=CARTESIAN_POINT ( 'NONE',  ( -40.00000000000002842, 80.00000000000001421, 52.50000000000014921 ) ) ;
#17796=ORIENTED_EDGE ( 'NONE', *, *, #18426, .F. ) ;
#17807=VERTEX_POINT ( 'NONE', #28507 ) ;
#17826=ORIENTED_EDGE ( 'NONE', *, *, #22358, .T. ) ;
#17840=FACE_OUTER_BOUND ( 'NONE', #11281, .T. ) ;
#17855=EDGE_CURVE ( 'NONE', #20591, #15313, #13752, .T. ) ;
#17861=DIRECTION ( 'NONE',  ( -1.000000000000000000, 0.000000000000000000, 0.000000000000000000 ) ) ;
#17874=CARTESIAN_POINT ( 'NONE',  ( -50.00000000000000000, -70.00000000000000000, 59.49999999999999289 ) ) ;
#17880=AXIS2_PLACEMENT_3D ( 'NONE', #390, #19421, #28940 ) ;
#17896=ORIENTED_EDGE ( 'NONE', *, *, #5222, .T. ) ;
#17903=CARTESIAN_POINT ( 'NONE',  ( -40.00000000000002842, 90.00000000000001421, 22.49999999999983302 ) ) ;
#17906=EDGE_LOOP ( 'NONE', ( #25562, #26599, #19153, #6833, #9966, #25437 ) ) ;
#17918=LINE ( 'NONE', #15561, #4318 ) ;
#17924=EDGE_CURVE ( 'NONE', #11277, #26276, #29278, .T. ) ;
#17945=CARTESIAN_POINT ( 'NONE',  ( 52.16608720827707657, -36.86186943028246787, 97.07879600563551037 ) ) ;
#17955=ORIENTED_EDGE ( 'NONE', *, *, #19143, .T. ) ;
#17960=CARTESIAN_POINT ( 'NONE',  ( -40.00000000000002842, 80.00000000000001421, 52.50000000000014921 ) ) ;
#17964=ADVANCED_FACE ( 'NONE', ( #14924 ), #9270, .T. ) ;
#17971=EDGE_LOOP ( 'NONE', ( #8276, #11916, #29489, #1811 ) ) ;
#17983=ORIENTED_EDGE ( 'NONE', *, *, #17361, .F. ) ;
#18000=CARTESIAN_POINT ( 'NONE',  ( -40.00000000000002842, 90.00000000000001421, 52.50000000000014921 ) ) ;
#18002=LINE ( 'NONE', #30145, #29685 ) ;
#18004=ADVANCED_FACE ( 'NONE', ( #5105 ), #5875, .T. ) ;
#18024=DIRECTION ( 'NONE',  ( -1.000000000000000000, -0.000000000000000000, 0.000000000000000000 ) ) ;
#18032=EDGE_LOOP ( 'NONE', ( #22975, #6196, #23744, #27995 ) ) ;
#18035=CARTESIAN_POINT ( 'NONE',  ( -43.01137460125430323, 68.74210893030173963, 12.95891939259967529 ) ) ;
#18037=CARTESIAN_POINT ( 'NONE',  ( -4.163336342344337027E-14, 1.387778780781445676E-14, 67.49999999999997158 ) ) ;
#18042=CARTESIAN_POINT ( 'NONE',  ( -7.075845757273814415E-16, 80.00000000000000000, 15.49999999999998757 ) ) ;
#18064=EDGE_CURVE ( 'NONE', #15359, #5466, #10293, .T. ) ;
#18070=DIRECTION ( 'NONE',  ( 0.000000000000000000, 0.000000000000000000, 1.000000000000000000 ) ) ;
#18087=DIRECTION ( 'NONE',  ( 1.000000000000000000, 0.000000000000000000, 0.000000000000000000 ) ) ;
#18101=EDGE_CURVE ( 'NONE', #7391, #23685, #1349, .T. ) ;
#18110=ORIENTED_EDGE ( 'NONE', *, *, #13569, .F. ) ;
#18118=DIRECTION ( 'NONE',  ( -0.000000000000000000, -0.000000000000000000, 1.000000000000000000 ) ) ;
#18135=EDGE_CURVE ( 'NONE', #30732, #5139, #5715, .T. ) ;
#18142=CARTESIAN_POINT ( 'NONE',  ( -70.00000000000000000, -65.00000000000000000, 12.49999999999999112 ) ) ;
#18143=EDGE_CURVE ( 'NONE', #15984, #22640, #24213, .T. ) ;
#18162=CARTESIAN_POINT ( 'NONE',  ( -50.00000000000000000, 90.00000000000001421, 52.49999999999999289 ) ) ;
#18172=ADVANCED_FACE ( 'NONE', ( #12543 ), #14266, .F. ) ;
#18186=DIRECTION ( 'NONE',  ( 1.000000000000000000, 0.000000000000000000, -0.000000000000000000 ) ) ;
#18202=EDGE_CURVE ( 'NONE', #228, #25790, #29995, .T. ) ;
#18204=DIRECTION ( 'NONE',  ( 0.000000000000000000, 0.000000000000000000, -1.000000000000000000 ) ) ;
#18212=LINE ( 'NONE', #8854, #2391 ) ;
#18233=CARTESIAN_POINT ( 'NONE',  ( 48.60441976126723773, 69.95499445371133618, 17.35986660046888019 ) ) ;
#18238=VECTOR ( 'NONE', #25421, 1000.000000000000000 ) ;
#18260=DIRECTION ( 'NONE',  ( 0.000000000000000000, 1.000000000000000000, 0.000000000000000000 ) ) ;
#18262=ORIENTED_EDGE ( 'NONE', *, *, #9947, .F. ) ;
#18265=DIRECTION ( 'NONE',  ( 0.000000000000000000, 0.000000000000000000, 1.000000000000000000 ) ) ;
#18269=CARTESIAN_POINT ( 'NONE',  ( 4.510281037539698445E-13, -4.926614671774132148E-13, 77.49999999999998579 ) ) ;
#18300=CARTESIAN_POINT ( 'NONE',  ( 52.16608720827707657, 36.86186943028246787, 97.07879600563551037 ) ) ;
#18307=ADVANCED_FACE ( 'NONE', ( #17840 ), #8630, .F. ) ;
#18317=EDGE_LOOP ( 'NONE', ( #300, #19299, #8282, #24901 ) ) ;
#18328=DIRECTION ( 'NONE',  ( 0.000000000000000000, 0.000000000000000000, -1.000000000000000000 ) ) ;
#18336=EDGE_CURVE ( 'NONE', #8546, #9249, #20246, .T. ) ;
#18337=AXIS2_PLACEMENT_3D ( 'NONE', #15664, #25029, #6007 ) ;
#18352=EDGE_CURVE ( 'NONE', #10409, #20585, #7040, .T. ) ;
#18362=EDGE_CURVE ( 'NONE', #20591, #27348, #20919, .T. ) ;
#18366=DIRECTION ( 'NONE',  ( 0.000000000000000000, 0.000000000000000000, -1.000000000000000000 ) ) ;
#18404=ORIENTED_EDGE ( 'NONE', *, *, #13774, .F. ) ;
#18412=ORIENTED_EDGE ( 'NONE', *, *, #6085, .T. ) ;
#18419=PLANE ( 'NONE',  #21898 ) ;
#18426=EDGE_CURVE ( 'NONE', #16566, #20079, #20981, .T. ) ;
#18459=CARTESIAN_POINT ( 'NONE',  ( 69.99999999999998579, -70.00000000000000000, 12.49999999999999112 ) ) ;
#18465=EDGE_LOOP ( 'NONE', ( #4783, #19162, #24919 ) ) ;
#18507=ORIENTED_EDGE ( 'NONE', *, *, #2498, .T. ) ;
#18520=CARTESIAN_POINT ( 'NONE',  ( -50.00000000000000000, 87.00000000000001421, 22.49999999999999289 ) ) ;
#18521=ORIENTED_EDGE ( 'NONE', *, *, #25806, .T. ) ;
#18543=EDGE_LOOP ( 'NONE', ( #6622, #23823, #1747, #20828 ) ) ;
#18554=EDGE_LOOP ( 'NONE', ( #11044, #25716, #5628, #9754 ) ) ;
#18558=CARTESIAN_POINT ( 'NONE',  ( 37.16608720827707657, 65.00000000000000000, 57.49999999999999289 ) ) ;
#18563=EDGE_CURVE ( 'NONE', #12285, #20725, #24109, .T. ) ;
#18574=CARTESIAN_POINT ( 'NONE',  ( -50.00000000000000000, 50.00000000000000000, 97.07879600563551037 ) ) ;
#18582=DIRECTION ( 'NONE',  ( 0.000000000000000000, 1.000000000000000000, -0.000000000000000000 ) ) ;
#18602=CARTESIAN_POINT ( 'NONE',  ( -4.163336342344337027E-14, 1.387778780781445676E-14, 67.49999999999997158 ) ) ;
#18616=DIRECTION ( 'NONE',  ( -0.000000000000000000, 1.000000000000000000, 0.000000000000000000 ) ) ;
#18619=DIRECTION ( 'NONE',  ( 0.000000000000000000, 0.000000000000000000, 1.000000000000000000 ) ) ;
#18641=CARTESIAN_POINT ( 'NONE',  ( -52.16608720827707657, 51.86186943028246787, 12.49999999999998401 ) ) ;
#18651=DIRECTION ( 'NONE',  ( 0.000000000000000000, 0.000000000000000000, 1.000000000000000000 ) ) ;
#18661=ORIENTED_EDGE ( 'NONE', *, *, #15485, .T. ) ;
#18675=CARTESIAN_POINT ( 'NONE',  ( 37.99999999999999289, 80.00000000000000000, 27.08257569495583184 ) ) ;
#18687=EDGE_CURVE ( 'NONE', #20672, #10252, #26254, .T. ) ;
#18691=VECTOR ( 'NONE', #26845, 1000.000000000000000 ) ;
#18693=ORIENTED_EDGE ( 'NONE', *, *, #7108, .T. ) ;
#18695=DIRECTION ( 'NONE',  ( 0.000000000000000000, 0.000000000000000000, 1.000000000000000000 ) ) ;
#18699=ADVANCED_FACE ( 'NONE', ( #24571 ), #1189, .T. ) ;
#18701=ORIENTED_EDGE ( 'NONE', *, *, #1327, .F. ) ;
#18745=B_SPLINE_CURVE_WITH_KNOTS ( 'NONE', 3,
 ( #30677, #26019, #25707, #25867, #23968, #21012, #16353, #4336, #23363, #7294, #16807, #26322, #11668, #2615 ),
 .UNSPECIFIED., .F., .F.,
 ( 4, 2, 2, 2, 2, 2, 4 ),
 ( 0.008361799641757327456, 0.009326569779210591715, 0.01029133991666385597, 0.01222088019157035327, 0.01318565032902361579, 0.01415042046647687832, 0.01607996074138338602 ),
 .UNSPECIFIED. ) ;
#18779=AXIS2_PLACEMENT_3D ( 'NONE', #14282, #24270, #19134 ) ;
#18786=AXIS2_PLACEMENT_3D ( 'NONE', #9237, #28273, #6898 ) ;
#18788=CARTESIAN_POINT ( 'NONE',  ( -4.163336342344337027E-14, 1.387778780781445676E-14, 67.49999999999997158 ) ) ;
#18795=ORIENTED_EDGE ( 'NONE', *, *, #29004, .T. ) ;
#18796=EDGE_CURVE ( 'NONE', #14360, #28974, #11164, .T. ) ;
#18798=CIRCLE ( 'NONE', #1369, 15.00000000000000000 ) ;
#18807=VECTOR ( 'NONE', #24953, 1000.000000000000000 ) ;
#18823=AXIS2_PLACEMENT_3D ( 'NONE', #18037, #27403, #10698 ) ;
#18824=DIRECTION ( 'NONE',  ( -1.000000000000000000, 0.000000000000000000, 0.000000000000000000 ) ) ;
#18826=EDGE_LOOP ( 'NONE', ( #185, #13148 ) ) ;
#18827=DIRECTION ( 'NONE',  ( -1.982541115402065356E-16, 0.000000000000000000, 1.000000000000000000 ) ) ;
#18844=CIRCLE ( 'NONE', #29303, 37.99999999999933920 ) ;
#18879=DIRECTION ( 'NONE',  ( -0.000000000000000000, -0.000000000000000000, -1.000000000000000000 ) ) ;
#18882=EDGE_LOOP ( 'NONE', ( #3944, #13504, #23093, #3422 ) ) ;
#18896=FACE_OUTER_BOUND ( 'NONE', #1418, .T. ) ;
#18897=CARTESIAN_POINT ( 'NONE',  ( 39.99999999999998579, 67.32050807568877815, 12.49999999999999112 ) ) ;
#18926=CARTESIAN_POINT ( 'NONE',  ( 37.16608720827707657, -65.00000000000000000, 57.49999999999999289 ) ) ;
#18932=CARTESIAN_POINT ( 'NONE',  ( -52.16608720827707657, -36.86186943028246787, 12.49999999999999112 ) ) ;
#18946=EDGE_CURVE ( 'NONE', #24152, #7862, #21756, .T. ) ;
#18952=EDGE_CURVE ( 'NONE', #509, #25203, #20768, .T. ) ;
#18968=DIRECTION ( 'NONE',  ( 0.000000000000000000, 0.000000000000000000, -1.000000000000000000 ) ) ;
#18979=EDGE_CURVE ( 'NONE', #27312, #12499, #7343, .T. ) ;
#18987=EDGE_LOOP ( 'NONE', ( #20258, #6673 ) ) ;
#18996=VERTEX_POINT ( 'NONE', #1463 ) ;
#18999=ORIENTED_EDGE ( 'NONE', *, *, #18352, .F. ) ;
#19028=ORIENTED_EDGE ( 'NONE', *, *, #2958, .T. ) ;
#19034=DIRECTION ( 'NONE',  ( -0.000000000000000000, -0.000000000000000000, 1.000000000000000000 ) ) ;
#19047=ORIENTED_EDGE ( 'NONE', *, *, #7080, .T. ) ;
#19059=VERTEX_POINT ( 'NONE', #8491 ) ;
#19060=LINE ( 'NONE', #26399, #17545 ) ;
#19066=AXIS2_PLACEMENT_3D ( 'NONE', #26589, #1837, #9018 ) ;
#19106=FACE_OUTER_BOUND ( 'NONE', #23413, .T. ) ;
#19111=CYLINDRICAL_SURFACE ( 'NONE', #17880, 50.00000000000000000 ) ;
#19119=VERTEX_POINT ( 'NONE', #10892 ) ;
#19120=VECTOR ( 'NONE', #10996, 1000.000000000000000 ) ;
#19134=DIRECTION ( 'NONE',  ( 0.000000000000000000, -0.000000000000000000, 1.000000000000000000 ) ) ;
#19143=EDGE_CURVE ( 'NONE', #19850, #13279, #19314, .T. ) ;
#19149=CIRCLE ( 'NONE', #14187, 6.999999999999999112 ) ;
#19152=LINE ( 'NONE', #28197, #10379 ) ;
#19153=ORIENTED_EDGE ( 'NONE', *, *, #10885, .F. ) ;
#19155=CARTESIAN_POINT ( 'NONE',  ( 49.99999999999998579, -67.00000000000000000, 59.49999999999999289 ) ) ;
#19161=AXIS2_PLACEMENT_3D ( 'NONE', #14734, #5539, #7426 ) ;
#19162=ORIENTED_EDGE ( 'NONE', *, *, #10765, .T. ) ;
#19174=LINE ( 'NONE', #12162, #28749 ) ;
#19176=ORIENTED_EDGE ( 'NONE', *, *, #20682, .T. ) ;
#19202=ORIENTED_EDGE ( 'NONE', *, *, #27367, .F. ) ;
#19214=VECTOR ( 'NONE', #21866, 1000.000000000000000 ) ;
#19244=TOROIDAL_SURFACE ( 'NONE', #27225, 7.000000000000000000, 3.000000000000000000 ) ;
#19245=CARTESIAN_POINT ( 'NONE',  ( -37.16608720827707657, 65.00000000000000000, 97.07879600563551037 ) ) ;
#19263=DIRECTION ( 'NONE',  ( 1.982541115402065110E-16, 0.000000000000000000, -1.000000000000000000 ) ) ;
#19271=CIRCLE ( 'NONE', #29739, 5.000000000000004441 ) ;
#19273=DIRECTION ( 'NONE',  ( 0.000000000000000000, 0.000000000000000000, -1.000000000000000000 ) ) ;
#19299=ORIENTED_EDGE ( 'NONE', *, *, #16012, .T. ) ;
#19314=CIRCLE ( 'NONE', #30747, 4.999999999999997335 ) ;
#19317=VERTEX_POINT ( 'NONE', #2129 ) ;
#19322=CIRCLE ( 'NONE', #8387, 3.000000000000002665 ) ;
#19359=AXIS2_PLACEMENT_3D ( 'NONE', #6190, #15691, #3851 ) ;
#19389=CARTESIAN_POINT ( 'NONE',  ( -40.00000000000000000, 67.32050807568877815, 12.49999999999999112 ) ) ;
#19391=ORIENTED_EDGE ( 'NONE', *, *, #381, .T. ) ;
#19404=CARTESIAN_POINT ( 'NONE',  ( 39.99999999999998579, 80.00000000000001421, 52.49999999999999289 ) ) ;
#19409=CIRCLE ( 'NONE', #11446, 7.500000000000013323 ) ;
#19410=DIRECTION ( 'NONE',  ( 0.000000000000000000, 0.000000000000000000, 1.000000000000000000 ) ) ;
#19417=ORIENTED_EDGE ( 'NONE', *, *, #22948, .F. ) ;
#19418=VERTEX_POINT ( 'NONE', #20850 ) ;
#19421=DIRECTION ( 'NONE',  ( -0.000000000000000000, -0.000000000000000000, -1.000000000000000000 ) ) ;
#19422=CARTESIAN_POINT ( 'NONE',  ( 37.16608720827707657, 65.00000000000000000, 12.49999999999999112 ) ) ;
#19429=CYLINDRICAL_SURFACE ( 'NONE', #12754, 5.000000000000004441 ) ;
#19430=AXIS2_PLACEMENT_3D ( 'NONE', #3848, #11024, #24907 ) ;
#19433=ORIENTED_EDGE ( 'NONE', *, *, #18336, .F. ) ;
#19440=CARTESIAN_POINT ( 'NONE',  ( -42.49999999999998579, -50.00000000000000000, 97.07879600563551037 ) ) ;
#19454=CARTESIAN_POINT ( 'NONE',  ( -29.99999999999933209, 1.755172820525642916E-14, 77.49999999999998579 ) ) ;
#19467=VERTEX_POINT ( 'NONE', #2449 ) ;
#19484=PLANE ( 'NONE',  #10772 ) ;
#19497=ADVANCED_FACE ( 'NONE', ( #8201 ), #27394, .T. ) ;
#19507=ADVANCED_FACE ( 'NONE', ( #27226 ), #3874, .T. ) ;
#19523=CARTESIAN_POINT ( 'NONE',  ( 0.000000000000000000, 80.00000000000000000, 50.49999999999998579 ) ) ;
#19531=EDGE_CURVE ( 'NONE', #5009, #24948, #15521, .T. ) ;
#19547=EDGE_LOOP ( 'NONE', ( #26440, #2896, #21015, #25758 ) ) ;
#19552=CARTESIAN_POINT ( 'NONE',  ( 39.99999999999998579, 80.00000000000001421, 47.49999999999999289 ) ) ;
#19570=EDGE_CURVE ( 'NONE', #20897, #23537, #7854, .T. ) ;
#19577=CARTESIAN_POINT ( 'NONE',  ( 0.000000000000000000, 80.00000000000000000, 50.49999999999998579 ) ) ;
#19583=ORIENTED_EDGE ( 'NONE', *, *, #29410, .F. ) ;
#19585=CIRCLE ( 'NONE', #1151, 45.00000000000000711 ) ;
#19586=VECTOR ( 'NONE', #5841, 1000.000000000000000 ) ;
#19594=CARTESIAN_POINT ( 'NONE',  ( -47.00000000000000000, 90.00000000000001421, 52.49999999999999289 ) ) ;
#19603=ORIENTED_EDGE ( 'NONE', *, *, #10180, .F. ) ;
#19619=DIRECTION ( 'NONE',  ( -1.000000000000000000, 0.000000000000000000, 0.000000000000000000 ) ) ;
#19624=FACE_OUTER_BOUND ( 'NONE', #28730, .T. ) ;
#19629=ORIENTED_EDGE ( 'NONE', *, *, #7108, .F. ) ;
#19632=CARTESIAN_POINT ( 'NONE',  ( -4.163336342344337027E-14, 1.387778780781445676E-14, 92.49999999999998579 ) ) ;
#19642=ADVANCED_FACE ( 'NONE', ( #3528, #20047, #5551, #20363, #10688, #10541 ), #707, .F. ) ;
#19648=VERTEX_POINT ( 'NONE', #5701 ) ;
#19671=CARTESIAN_POINT ( 'NONE',  ( -45.40481444351987506, 69.10337004759016111, 60.91566614034201876 ) ) ;
#19686=CARTESIAN_POINT ( 'NONE',  ( -70.00000000000000000, -70.00000000000000000, 12.49999999999999112 ) ) ;
#19704=ADVANCED_FACE ( 'NONE', ( #4440 ), #13951, .F. ) ;
#19707=EDGE_CURVE ( 'NONE', #25448, #30732, #14831, .T. ) ;
#19724=AXIS2_PLACEMENT_3D ( 'NONE', #23673, #2485, #12001 ) ;
#19725=LINE ( 'NONE', #10214, #6707 ) ;
#19729=CARTESIAN_POINT ( 'NONE',  ( -4.163336342344337027E-14, 1.387778780781445676E-14, 77.49999999999998579 ) ) ;
#19734=ADVANCED_FACE ( 'NONE', ( #1646 ), #2085, .T. ) ;
#19736=DIRECTION ( 'NONE',  ( -1.000000000000000000, 0.000000000000000000, -0.000000000000000000 ) ) ;
#19749=CARTESIAN_POINT ( 'NONE',  ( 49.99999999999998579, -50.00000000000000000, 59.49999999999999289 ) ) ;
#19761=ORIENTED_EDGE ( 'NONE', *, *, #30551, .T. ) ;
#19770=CIRCLE ( 'NONE', #30721, 45.00000000000000711 ) ;
#19782=CIRCLE ( 'NONE', #22354, 4.999999999999997335 ) ;
#19798=DIRECTION ( 'NONE',  ( 0.000000000000000000, 1.000000000000000000, 0.000000000000000000 ) ) ;
#19800=CARTESIAN_POINT ( 'NONE',  ( -37.16608720827707657, 36.86186943028246787, 12.49999999999999112 ) ) ;
#19839=CIRCLE ( 'NONE', #12887, 7.500000000000013323 ) ;
#19850=VERTEX_POINT ( 'NONE', #6624 ) ;
#19891=LINE ( 'NONE', #26607, #25875 ) ;
#19895=ORIENTED_EDGE ( 'NONE', *, *, #5801, .T. ) ;
#19905=EDGE_CURVE ( 'NONE', #25203, #509, #22811, .T. ) ;
#19922=CIRCLE ( 'NONE', #4470, 20.00000000000000355 ) ;
#19932=ORIENTED_EDGE ( 'NONE', *, *, #10266, .T. ) ;
#19939=VECTOR ( 'NONE', #3167, 1000.000000000000000 ) ;
#19957=DIRECTION ( 'NONE',  ( 0.000000000000000000, 0.000000000000000000, -1.000000000000000000 ) ) ;
#19966=ORIENTED_EDGE ( 'NONE', *, *, #2882, .T. ) ;
#19972=ORIENTED_EDGE ( 'NONE', *, *, #6576, .T. ) ;
#19974=DIRECTION ( 'NONE',  ( -0.000000000000000000, 1.000000000000000000, -0.000000000000000000 ) ) ;
#19988=CARTESIAN_POINT ( 'NONE',  ( 44.92383873364811819, 68.80441998829734018, 61.21192490580749990 ) ) ;
#19998=EDGE_LOOP ( 'NONE', ( #13343, #12660, #11752, #11028 ) ) ;
#20007=ORIENTED_EDGE ( 'NONE', *, *, #23006, .T. ) ;
#20037=EDGE_CURVE ( 'NONE', #29034, #5009, #4241, .T. ) ;
#20038=ORIENTED_EDGE ( 'NONE', *, *, #482, .T. ) ;
#20046=DIRECTION ( 'NONE',  ( 0.000000000000000000, 1.000000000000000000, 0.000000000000000000 ) ) ;
#20047=FACE_BOUND ( 'NONE', #667, .T. ) ;
#20052=TOROIDAL_SURFACE ( 'NONE', #8622, 7.000000000000000000, 3.000000000000000000 ) ;
#20069=FACE_BOUND ( 'NONE', #3964, .T. ) ;
#20076=VECTOR ( 'NONE', #7006, 1000.000000000000000 ) ;
#20079=VERTEX_POINT ( 'NONE', #1616 ) ;
#20104=TOROIDAL_SURFACE ( 'NONE', #3680, 37.99999999999933920, 3.000000000000000000 ) ;
#20113=VERTEX_POINT ( 'NONE', #28568 ) ;
#20129=EDGE_LOOP ( 'NONE', ( #2373, #7205 ) ) ;
#20141=FACE_OUTER_BOUND ( 'NONE', #16379, .T. ) ;
#20189=ORIENTED_EDGE ( 'NONE', *, *, #6550, .F. ) ;
#20200=EDGE_CURVE ( 'NONE', #20533, #30406, #19770, .T. ) ;
#20201=DIRECTION ( 'NONE',  ( 0.000000000000000000, 0.000000000000000000, 1.000000000000000000 ) ) ;
#20229=DIRECTION ( 'NONE',  ( 0.000000000000000000, 1.000000000000000000, 0.000000000000000000 ) ) ;
#20234=ADVANCED_FACE ( 'NONE', ( #2828 ), #23881, .T. ) ;
#20246=CIRCLE ( 'NONE', #17266, 5.000000000000004441 ) ;
#20258=ORIENTED_EDGE ( 'NONE', *, *, #19905, .T. ) ;
#20267=VECTOR ( 'NONE', #26307, 1000.000000000000000 ) ;
#20282=AXIS2_PLACEMENT_3D ( 'NONE', #1238, #9279, #28322 ) ;
#20294=AXIS2_PLACEMENT_3D ( 'NONE', #10943, #29959, #4202 ) ;
#20298=CARTESIAN_POINT ( 'NONE',  ( 39.99999999999998579, 63.74772708486752038, 62.49999999999999289 ) ) ;
#20299=ORIENTED_EDGE ( 'NONE', *, *, #24422, .T. ) ;
#20304=DIRECTION ( 'NONE',  ( 0.000000000000000000, 0.000000000000000000, -1.000000000000000000 ) ) ;
#20305=CARTESIAN_POINT ( 'NONE',  ( -52.16608720827707657, -51.86186943028246787, 57.49999999999999289 ) ) ;
#20316=AXIS2_PLACEMENT_3D ( 'NONE', #4140, #3837, #13363 ) ;
#20330=DIRECTION ( 'NONE',  ( -0.000000000000000000, -0.000000000000000000, 1.000000000000000000 ) ) ;
#20334=ORIENTED_EDGE ( 'NONE', *, *, #18362, .T. ) ;
#20343=CARTESIAN_POINT ( 'NONE',  ( -7.483314773547907528, 75.00000000000001421, 50.49999999999998579 ) ) ;
#20349=EDGE_CURVE ( 'NONE', #12825, #15108, #26171, .T. ) ;
#20363=FACE_BOUND ( 'NONE', #17790, .T. ) ;
#20377=ORIENTED_EDGE ( 'NONE', *, *, #29964, .T. ) ;
#20380=CARTESIAN_POINT ( 'NONE',  ( 0.000000000000000000, 80.00000000000000000, 50.49999999999998579 ) ) ;
#20381=CARTESIAN_POINT ( 'NONE',  ( -50.00000000000000000, -50.00000000000000000, 12.49999999999999112 ) ) ;
#20384=( NAMED_UNIT ( * ) SI_UNIT ( $, .STERADIAN. ) SOLID_ANGLE_UNIT ( ) );
#20394=CARTESIAN_POINT ( 'NONE',  ( -2.081668171172168513E-14, 90.00000000000001421, 52.49999999999999289 ) ) ;
#20405=DIRECTION ( 'NONE',  ( -1.000000000000000000, 0.000000000000000000, 0.000000000000000000 ) ) ;
#20417=CARTESIAN_POINT ( 'NONE',  ( 41.18405171698749001, 67.96430988548668495, 12.55145055161026058 ) ) ;
#20426=ORIENTED_EDGE ( 'NONE', *, *, #9051, .F. ) ;
#20432=ORIENTED_EDGE ( 'NONE', *, *, #23131, .T. ) ;
#20456=CARTESIAN_POINT ( 'NONE',  ( 64.99999999999998579, -36.86186943028246787, 57.49999999999999289 ) ) ;
#20462=ORIENTED_EDGE ( 'NONE', *, *, #3661, .F. ) ;
#20468=ORIENTED_EDGE ( 'NONE', *, *, #10964, .T. ) ;
#20473=ORIENTED_EDGE ( 'NONE', *, *, #12472, .T. ) ;
#20487=CYLINDRICAL_SURFACE ( 'NONE', #10577, 10.00000000000000178 ) ;
#20490=DIRECTION ( 'NONE',  ( 0.000000000000000000, 0.000000000000000000, -1.000000000000000000 ) ) ;
#20492=DIRECTION ( 'NONE',  ( -0.000000000000000000, 1.000000000000000000, -0.000000000000000000 ) ) ;
#20501=AXIS2_PLACEMENT_3D ( 'NONE', #12370, #17038, #2849 ) ;
#20507=AXIS2_PLACEMENT_3D ( 'NONE', #29261, #12894, #13043 ) ;
#20533=VERTEX_POINT ( 'NONE', #21916 ) ;
#20540=DIRECTION ( 'NONE',  ( -1.000000000000000000, 0.000000000000000000, -1.982541115402065356E-16 ) ) ;
#20557=VERTEX_POINT ( 'NONE', #3355 ) ;
#20558=EDGE_LOOP ( 'NONE', ( #11448, #29809, #6479, #16008 ) ) ;
#20559=CARTESIAN_POINT ( 'NONE',  ( 43.30651650232057648, 68.84932239039000024, 13.05702333277023719 ) ) ;
#20576=AXIS2_PLACEMENT_3D ( 'NONE', #21322, #30535, #30840 ) ;
#20583=DIRECTION ( 'NONE',  ( 0.000000000000000000, 0.000000000000000000, 1.000000000000000000 ) ) ;
#20585=VERTEX_POINT ( 'NONE', #10217 ) ;
#20591=VERTEX_POINT ( 'NONE', #29252 ) ;
#20592=ORIENTED_EDGE ( 'NONE', *, *, #14508, .T. ) ;
#20623=DIRECTION ( 'NONE',  ( -0.000000000000000000, -1.000000000000000000, -0.000000000000000000 ) ) ;
#20639=EDGE_LOOP ( 'NONE', ( #19047, #21629, #13047, #30408, #19391, #3971, #9945, #24435, #5393, #22264, #24197, #12988, #8527 ) ) ;
#20663=CARTESIAN_POINT ( 'NONE',  ( -48.93034346171027238, 69.97313033977476948, 17.95007235832140324 ) ) ;
#20671=ORIENTED_EDGE ( 'NONE', *, *, #2489, .F. ) ;
#20672=VERTEX_POINT ( 'NONE', #13906 ) ;
#20675=DIRECTION ( 'NONE',  ( -1.224646799147353207E-16, 1.000000000000000000, 0.000000000000000000 ) ) ;
#20679=EDGE_CURVE ( 'NONE', #30078, #3647, #23702, .T. ) ;
#20682=EDGE_CURVE ( 'NONE', #1222, #21772, #11424, .T. ) ;
#20683=CARTESIAN_POINT ( 'NONE',  ( -40.00000000000002842, 80.00000000000001421, 22.49999999999983302 ) ) ;
#20712=FACE_BOUND ( 'NONE', #30098, .T. ) ;
#20720=ORIENTED_EDGE ( 'NONE', *, *, #27366, .T. ) ;
#20725=VERTEX_POINT ( 'NONE', #8933 ) ;
#20743=AXIS2_PLACEMENT_3D ( 'NONE', #12351, #9688, #2524 ) ;
#20768=CIRCLE ( 'NONE', #23750, 34.99999999999933920 ) ;
#20790=VECTOR ( 'NONE', #17642, 1000.000000000000000 ) ;
#20791=ADVANCED_FACE ( 'NONE', ( #16095 ), #13618, .F. ) ;
#20802=VERTEX_POINT ( 'NONE', #25617 ) ;
#20816=FACE_BOUND ( 'NONE', #18826, .T. ) ;
#20817=CARTESIAN_POINT ( 'NONE',  ( -48.03319056991080771, 69.90398198426727561, 16.53503636252214193 ) ) ;
#20828=ORIENTED_EDGE ( 'NONE', *, *, #207, .F. ) ;
#20834=ORIENTED_EDGE ( 'NONE', *, *, #10197, .F. ) ;
#20842=CIRCLE ( 'NONE', #6408, 7.500000000000013323 ) ;
#20850=CARTESIAN_POINT ( 'NONE',  ( -47.14142842854255377, 69.79466010243307039, 59.50000000000029843 ) ) ;
#20862=EDGE_CURVE ( 'NONE', #10409, #12881, #25109, .T. ) ;
#20874=DIRECTION ( 'NONE',  ( 0.000000000000000000, 0.000000000000000000, 1.000000000000000000 ) ) ;
#20876=CARTESIAN_POINT ( 'NONE',  ( -37.16608720827707657, 36.86186943028246787, 57.49999999999999289 ) ) ;
#20882=CARTESIAN_POINT ( 'NONE',  ( -70.00000000000000000, 65.00000000000000000, 12.49999999999999112 ) ) ;
#20884=VECTOR ( 'NONE', #25135, 1000.000000000000000 ) ;
#20886=CYLINDRICAL_SURFACE ( 'NONE', #27090, 4.999999999999997335 ) ;
#20893=CYLINDRICAL_SURFACE ( 'NONE', #24193, 7.500000000000013323 ) ;
#20897=VERTEX_POINT ( 'NONE', #5774 ) ;
#20908=VECTOR ( 'NONE', #18968, 1000.000000000000000 ) ;
#20910=DIRECTION ( 'NONE',  ( 0.000000000000000000, 1.000000000000000000, 0.000000000000000000 ) ) ;
#20912=ORIENTED_EDGE ( 'NONE', *, *, #25196, .T. ) ;
#20919=LINE ( 'NONE', #21, #8810 ) ;
#20942=EDGE_LOOP ( 'NONE', ( #1372, #27679, #20949, #18404 ) ) ;
#20947=DIRECTION ( 'NONE',  ( -0.000000000000000000, -0.000000000000000000, 1.000000000000000000 ) ) ;
#20949=ORIENTED_EDGE ( 'NONE', *, *, #9543, .T. ) ;
#20953=DIRECTION ( 'NONE',  ( -0.000000000000000000, -1.000000000000000000, -0.000000000000000000 ) ) ;
#20954=CYLINDRICAL_SURFACE ( 'NONE', #15118, 15.00000000000000000 ) ;
#20958=EDGE_CURVE ( 'NONE', #3050, #26039, #29335, .T. ) ;
#20963=DIRECTION ( 'NONE',  ( 0.000000000000000000, 0.000000000000000000, 1.000000000000000000 ) ) ;
#20964=EDGE_CURVE ( 'NONE', #15944, #19119, #22606, .T. ) ;
#20981=B_SPLINE_CURVE_WITH_KNOTS ( 'NONE', 3,
 ( #27963, #6590, #17326, #779, #14523, #14670, #28722, #26856, #29176, #7664, #7985, #2669 ),
 .UNSPECIFIED., .F., .F.,
 ( 4, 2, 2, 2, 2, 4 ),
 ( 0.000000000000000000, 0.001930342444571962182, 0.002895513666857931455, 0.003860684889143900511, 0.005791027333715810868, 0.007721369778287722092 ),
 .UNSPECIFIED. ) ;
#21003=DIRECTION ( 'NONE',  ( -1.000000000000000000, 0.000000000000000000, 0.000000000000000000 ) ) ;
#21007=CIRCLE ( 'NONE', #14543, 47.00000000000000000 ) ;
#21012=CARTESIAN_POINT ( 'NONE',  ( -48.71096830872563999, 69.96160472130995345, 57.45356189401062608 ) ) ;
#21014=DIRECTION ( 'NONE',  ( 1.000000000000000000, 0.000000000000000000, 0.000000000000000000 ) ) ;
#21015=ORIENTED_EDGE ( 'NONE', *, *, #13975, .T. ) ;
#21017=DIRECTION ( 'NONE',  ( -1.000000000000000000, 0.000000000000000000, 0.000000000000000000 ) ) ;
#21055=DIRECTION ( 'NONE',  ( 1.000000000000000000, 0.000000000000000000, 0.000000000000000000 ) ) ;
#21080=CARTESIAN_POINT ( 'NONE',  ( 39.99999999999998579, -0.000000000000000000, 22.49999999999999289 ) ) ;
#21104=EDGE_LOOP ( 'NONE', ( #20432, #23078, #11628, #1849, #7703, #11216, #25244 ) ) ;
#21138=ORIENTED_EDGE ( 'NONE', *, *, #23671, .F. ) ;
#21147=CARTESIAN_POINT ( 'NONE',  ( -47.00000000000000000, 87.00000000000001421, 0.000000000000000000 ) ) ;
#21178=CARTESIAN_POINT ( 'NONE',  ( -70.00000000000000000, -50.00000000000000000, 12.49999999999999112 ) ) ;
#21187=ORIENTED_EDGE ( 'NONE', *, *, #20862, .F. ) ;
#21191=CARTESIAN_POINT ( 'NONE',  ( 0.000000000000000000, 80.00000000000000000, 0.000000000000000000 ) ) ;
#21207=AXIS2_PLACEMENT_3D ( 'NONE', #11434, #20623, #27819 ) ;
#21241=CARTESIAN_POINT ( 'NONE',  ( -50.00000000000000000, 50.00000000000000000, 12.49999999999999112 ) ) ;
#21253=AXIS2_PLACEMENT_3D ( 'NONE', #1034, #3212, #14914 ) ;
#21264=ORIENTED_EDGE ( 'NONE', *, *, #29414, .F. ) ;
#21266=AXIS2_PLACEMENT_3D ( 'NONE', #7199, #16712, #327 ) ;
#21285=LINE ( 'NONE', #7109, #1688 ) ;
#21286=ORIENTED_EDGE ( 'NONE', *, *, #6448, .F. ) ;
#21288=VECTOR ( 'NONE', #22038, 1000.000000000000000 ) ;
#21295=DIRECTION ( 'NONE',  ( 0.000000000000000000, 0.000000000000000000, -1.000000000000000000 ) ) ;
#21300=DIRECTION ( 'NONE',  ( -0.000000000000000000, -1.000000000000000000, -0.000000000000000000 ) ) ;
#21309=FACE_OUTER_BOUND ( 'NONE', #24839, .T. ) ;
#21313=CARTESIAN_POINT ( 'NONE',  ( 4.510281037539698445E-13, -4.926614671774132148E-13, 65.49999999999998579 ) ) ;
#21322=CARTESIAN_POINT ( 'NONE',  ( -37.99999999999933920, 4.653657836759860688E-15, 85.49999999999998579 ) ) ;
#21350=EDGE_CURVE ( 'NONE', #17431, #8898, #18212, .T. ) ;
#21364=DIRECTION ( 'NONE',  ( 0.000000000000000000, -0.000000000000000000, -1.000000000000000000 ) ) ;
#21378=VERTEX_POINT ( 'NONE', #27887 ) ;
#21394=ADVANCED_FACE ( 'NONE', ( #9009 ), #16020, .T. ) ;
#21397=DIRECTION ( 'NONE',  ( 0.000000000000000000, 0.000000000000000000, 1.000000000000000000 ) ) ;
#21406=ADVANCED_FACE ( 'NONE', ( #13988 ), #23342, .T. ) ;
#21412=LINE ( 'NONE', #19686, #14925 ) ;
#21414=ORIENTED_EDGE ( 'NONE', *, *, #12862, .F. ) ;
#21415=CARTESIAN_POINT ( 'NONE',  ( -40.00000000000002842, 90.00000000000001421, 17.49999999999982947 ) ) ;
#21420=ADVANCED_FACE ( 'NONE', ( #30653 ), #9301, .F. ) ;
#21433=CARTESIAN_POINT ( 'NONE',  ( -52.16608720827707657, -51.86186943028246787, 97.07879600563551037 ) ) ;
#21450=ORIENTED_EDGE ( 'NONE', *, *, #17433, .F. ) ;
#21496=DIRECTION ( 'NONE',  ( 0.000000000000000000, 0.000000000000000000, 1.000000000000000000 ) ) ;
#21501=DIRECTION ( 'NONE',  ( 0.000000000000000000, 0.000000000000000000, -1.000000000000000000 ) ) ;
#21506=LINE ( 'NONE', #148, #6648 ) ;
#21511=CARTESIAN_POINT ( 'NONE',  ( 64.99999999999998579, -70.00000000000000000, 12.49999999999999112 ) ) ;
#21524=CARTESIAN_POINT ( 'NONE',  ( 39.99999999999996447, 90.00000000000001421, 59.49999999999999289 ) ) ;
#21530=DIRECTION ( 'NONE',  ( -0.000000000000000000, -0.000000000000000000, -1.000000000000000000 ) ) ;
#21541=DIRECTION ( 'NONE',  ( 0.000000000000000000, -1.000000000000000000, 0.000000000000000000 ) ) ;
#21546=LINE ( 'NONE', #12362, #19214 ) ;
#21570=EDGE_CURVE ( 'NONE', #20802, #29075, #406, .T. ) ;
#21581=CARTESIAN_POINT ( 'NONE',  ( 34.99999999999933920, 4.286263797015655244E-15, 92.49999999999998579 ) ) ;
#21593=ORIENTED_EDGE ( 'NONE', *, *, #30132, .T. ) ;
#21604=EDGE_LOOP ( 'NONE', ( #20377, #5612 ) ) ;
#21629=ORIENTED_EDGE ( 'NONE', *, *, #27155, .T. ) ;
#21636=DIRECTION ( 'NONE',  ( 1.982541115402065110E-16, 0.000000000000000000, -1.000000000000000000 ) ) ;
#21654=CARTESIAN_POINT ( 'NONE',  ( -52.16608720827707657, 36.86186943028246787, 57.49999999999999289 ) ) ;
#21659=DIRECTION ( 'NONE',  ( 0.000000000000000000, 1.000000000000000000, 0.000000000000000000 ) ) ;
#21680=CARTESIAN_POINT ( 'NONE',  ( 4.510281037539698445E-13, -4.926614671774132148E-13, 82.49999999999998579 ) ) ;
#21682=VECTOR ( 'NONE', #8148, 1000.000000000000000 ) ;
#21706=ORIENTED_EDGE ( 'NONE', *, *, #14163, .T. ) ;
#21708=CARTESIAN_POINT ( 'NONE',  ( -40.00000000000000000, 90.00000000000001421, 22.49999999999999289 ) ) ;
#21716=CIRCLE ( 'NONE', #8295, 3.000000000000002665 ) ;
#21733=AXIS2_PLACEMENT_3D ( 'NONE', #3631, #13150, #1293 ) ;
#21751=LINE ( 'NONE', #19422, #17562 ) ;
#21753=CARTESIAN_POINT ( 'NONE',  ( 4.510281037539698445E-13, -4.926614671774132148E-13, 82.49999999999998579 ) ) ;
#21756=CIRCLE ( 'NONE', #10317, 20.00000000000000000 ) ;
#21771=VECTOR ( 'NONE', #18879, 1000.000000000000000 ) ;
#21772=VERTEX_POINT ( 'NONE', #3056 ) ;
#21775=AXIS2_PLACEMENT_3D ( 'NONE', #13278, #25117, #3757 ) ;
#21777=VECTOR ( 'NONE', #6584, 1000.000000000000000 ) ;
#21779=AXIS2_PLACEMENT_3D ( 'NONE', #10853, #25182, #29263 ) ;
#21788=ORIENTED_EDGE ( 'NONE', *, *, #28456, .F. ) ;
#21790=ORIENTED_EDGE ( 'NONE', *, *, #24422, .F. ) ;
#21805=VECTOR ( 'NONE', #5861, 1000.000000000000000 ) ;
#21824=CARTESIAN_POINT ( 'NONE',  ( -40.00000000000000000, 87.00000000000001421, 62.49999999999999289 ) ) ;
#21838=LINE ( 'NONE', #9677, #18691 ) ;
#21839=CIRCLE ( 'NONE', #8412, 5.000000000000004441 ) ;
#21851=DIRECTION ( 'NONE',  ( 0.000000000000000000, -1.000000000000000000, 0.000000000000000000 ) ) ;
#21863=CARTESIAN_POINT ( 'NONE',  ( 52.16608720827707657, 36.86186943028246787, 57.49999999999999289 ) ) ;
#21866=DIRECTION ( 'NONE',  ( -1.000000000000000000, -0.000000000000000000, -0.000000000000000000 ) ) ;
#21876=ORIENTED_EDGE ( 'NONE', *, *, #18952, .F. ) ;
#21879=DIRECTION ( 'NONE',  ( 1.000000000000000000, 0.000000000000000000, 0.000000000000000000 ) ) ;
#21893=DIRECTION ( 'NONE',  ( 0.000000000000000000, 0.000000000000000000, -1.000000000000000000 ) ) ;
#21898=AXIS2_PLACEMENT_3D ( 'NONE', #20882, #30407, #11680 ) ;
#21908=FACE_OUTER_BOUND ( 'NONE', #1365, .T. ) ;
#21916=CARTESIAN_POINT ( 'NONE',  ( 45.00000000000045475, -4.871505565812501079E-13, 77.49999999999998579 ) ) ;
#21918=AXIS2_PLACEMENT_3D ( 'NONE', #6032, #3385, #12915 ) ;
#21938=DIRECTION ( 'NONE',  ( -1.000000000000000000, 0.000000000000000000, 0.000000000000000000 ) ) ;
#21939=CARTESIAN_POINT ( 'NONE',  ( 45.00000000000045475, -4.871505565812501079E-13, 57.49999999999999289 ) ) ;
#21941=EDGE_LOOP ( 'NONE', ( #23737, #8733, #7788, #12707, #20007, #29447, #4640, #28454, #8058, #17388, #747, #29803, #21706, #28926, #19895, #12755 ) ) ;
#21954=EDGE_LOOP ( 'NONE', ( #15782, #26833, #29721, #16591 ) ) ;
#21962=EDGE_CURVE ( 'NONE', #10235, #25178, #20842, .T. ) ;
#21969=CARTESIAN_POINT ( 'NONE',  ( -37.16608720827707657, 51.86186943028246787, 12.49999999999999112 ) ) ;
#21975=VECTOR ( 'NONE', #23155, 1000.000000000000000 ) ;
#21979=DIRECTION ( 'NONE',  ( 0.000000000000000000, -1.000000000000000000, 0.000000000000000000 ) ) ;
#21980=DIRECTION ( 'NONE',  ( 0.000000000000000000, 0.000000000000000000, 1.000000000000000000 ) ) ;
#21983=DIRECTION ( 'NONE',  ( -0.000000000000000000, -0.000000000000000000, 1.000000000000000000 ) ) ;
#21991=ORIENTED_EDGE ( 'NONE', *, *, #1524, .F. ) ;
#21999=DIRECTION ( 'NONE',  ( 0.000000000000000000, 0.000000000000000000, 1.000000000000000000 ) ) ;
#22010=CARTESIAN_POINT ( 'NONE',  ( 46.04937334709716623, 69.44700547456450579, 60.46534098734598928 ) ) ;
#22015=DIRECTION ( 'NONE',  ( 0.000000000000000000, 0.000000000000000000, 1.000000000000000000 ) ) ;
#22033=EDGE_LOOP ( 'NONE', ( #19583, #15219, #19028, #26996 ) ) ;
#22038=DIRECTION ( 'NONE',  ( -0.000000000000000000, 1.000000000000000000, -0.000000000000000000 ) ) ;
#22044=ORIENTED_EDGE ( 'NONE', *, *, #14496, .F. ) ;
#22045=DIRECTION ( 'NONE',  ( -1.000000000000000000, 0.000000000000000000, 0.000000000000000000 ) ) ;
#22061=DIRECTION ( 'NONE',  ( -0.000000000000000000, 1.000000000000000000, -0.000000000000000000 ) ) ;
#22073=DIRECTION ( 'NONE',  ( 0.000000000000000000, 0.000000000000000000, 1.000000000000000000 ) ) ;
#22079=LINE ( 'NONE', #27083, #839 ) ;
#22119=CARTESIAN_POINT ( 'NONE',  ( 37.16608720827707657, -36.86186943028246787, 97.07879600563551037 ) ) ;
#22140=EDGE_CURVE ( 'NONE', #4513, #2571, #2080, .T. ) ;
#22142=CARTESIAN_POINT ( 'NONE',  ( -50.00000000000000000, -50.00000000000000000, 12.49999999999999112 ) ) ;
#22144=EDGE_CURVE ( 'NONE', #10762, #4980, #10391, .T. ) ;
#22176=FACE_OUTER_BOUND ( 'NONE', #8685, .T. ) ;
#22177=DIRECTION ( 'NONE',  ( -0.000000000000000000, -0.000000000000000000, 1.000000000000000000 ) ) ;
#22184=AXIS2_PLACEMENT_3D ( 'NONE', #11712, #4689, #11421 ) ;
#22219=DIRECTION ( 'NONE',  ( 0.000000000000000000, 0.000000000000000000, 1.000000000000000000 ) ) ;
#22221=DIRECTION ( 'NONE',  ( 0.000000000000000000, 0.000000000000000000, -1.000000000000000000 ) ) ;
#22234=ORIENTED_EDGE ( 'NONE', *, *, #29756, .T. ) ;
#22235=DIRECTION ( 'NONE',  ( 0.000000000000000000, 1.000000000000000000, 0.000000000000000000 ) ) ;
#22243=CIRCLE ( 'NONE', #23716, 20.00000000000000000 ) ;
#22264=ORIENTED_EDGE ( 'NONE', *, *, #28051, .T. ) ;
#22284=EDGE_LOOP ( 'NONE', ( #12693, #8103, #15573, #16738, #25966, #3132 ) ) ;
#22293=DIRECTION ( 'NONE',  ( -1.000000000000000000, 0.000000000000000000, 0.000000000000000000 ) ) ;
#22314=ADVANCED_FACE ( 'NONE', ( #24956 ), #3594, .F. ) ;
#22322=DIRECTION ( 'NONE',  ( -0.000000000000000000, -0.000000000000000000, -1.000000000000000000 ) ) ;
#22326=PLANE ( 'NONE',  #24855 ) ;
#22334=CARTESIAN_POINT ( 'NONE',  ( 66.99999999999998579, 0.000000000000000000, 59.49999999999999289 ) ) ;
#22349=EDGE_CURVE ( 'NONE', #25448, #30732, #24124, .T. ) ;
#22354=AXIS2_PLACEMENT_3D ( 'NONE', #23763, #28616, #19410 ) ;
#22357=VECTOR ( 'NONE', #26155, 1000.000000000000000 ) ;
#22358=EDGE_CURVE ( 'NONE', #11642, #498, #23840, .T. ) ;
#22374=VERTEX_POINT ( 'NONE', #13067 ) ;
#22380=ORIENTED_EDGE ( 'NONE', *, *, #29410, .T. ) ;
#22389=DIRECTION ( 'NONE',  ( -0.000000000000000000, -0.000000000000000000, 1.000000000000000000 ) ) ;
#22397=CARTESIAN_POINT ( 'NONE',  ( 39.99999999999998579, 80.00000000000001421, 22.49999999999999289 ) ) ;
#22402=CARTESIAN_POINT ( 'NONE',  ( -65.00000000000000000, -70.00000000000000000, 12.49999999999999112 ) ) ;
#22406=LINE ( 'NONE', #28967, #26536 ) ;
#22408=ORIENTED_EDGE ( 'NONE', *, *, #13012, .T. ) ;
#22421=EDGE_LOOP ( 'NONE', ( #1016, #11385, #8939, #25989 ) ) ;
#22424=CARTESIAN_POINT ( 'NONE',  ( 39.99999999999998579, 80.00000000000001421, 52.49999999999999289 ) ) ;
#22458=CIRCLE ( 'NONE', #1551, 15.00000000000000000 ) ;
#22466=CARTESIAN_POINT ( 'NONE',  ( -40.00000000000000000, 87.00000000000001421, 15.49999999999998934 ) ) ;
#22472=CARTESIAN_POINT ( 'NONE',  ( -40.49689208720899813, 64.44504373098514804, 62.50000000000000000 ) ) ;
#22476=CYLINDRICAL_SURFACE ( 'NONE', #11637, 3.000000000000002665 ) ;
#22480=VECTOR ( 'NONE', #164, 1000.000000000000000 ) ;
#22485=ORIENTED_EDGE ( 'NONE', *, *, #10728, .T. ) ;
#22497=CARTESIAN_POINT ( 'NONE',  ( -40.00000000000002842, 80.00000000000001421, 47.50000000000014921 ) ) ;
#22505=DIRECTION ( 'NONE',  ( 0.000000000000000000, -1.000000000000000000, 0.000000000000000000 ) ) ;
#22508=CARTESIAN_POINT ( 'NONE',  ( -67.00000000000000000, 50.00000000000000000, 59.49999999999999289 ) ) ;
#22509=LINE ( 'NONE', #8510, #19586 ) ;
#22521=EDGE_CURVE ( 'NONE', #25063, #19467, #12918, .T. ) ;
#22527=LINE ( 'NONE', #17874, #4353 ) ;
#22536=VERTEX_POINT ( 'NONE', #23327 ) ;
#22543=CARTESIAN_POINT ( 'NONE',  ( 7.483314773547865784, 75.00000000000001421, 50.49999999999998579 ) ) ;
#22555=EDGE_CURVE ( 'NONE', #4126, #886, #6912, .T. ) ;
#22558=ORIENTED_EDGE ( 'NONE', *, *, #8811, .F. ) ;
#22568=FACE_BOUND ( 'NONE', #24756, .T. ) ;
#22573=ORIENTED_EDGE ( 'NONE', *, *, #17397, .T. ) ;
#22604=ORIENTED_EDGE ( 'NONE', *, *, #16117, .F. ) ;
#22606=LINE ( 'NONE', #17480, #9335 ) ;
#22608=ORIENTED_EDGE ( 'NONE', *, *, #9581, .F. ) ;
#22610=AXIS2_PLACEMENT_3D ( 'NONE', #26688, #5784, #15281 ) ;
#22625=CARTESIAN_POINT ( 'NONE',  ( 46.52886723831935711, 69.65281032693101793, 60.08552518507810447 ) ) ;
#22629=CYLINDRICAL_SURFACE ( 'NONE', #14118, 15.00000000000000000 ) ;
#22640=VERTEX_POINT ( 'NONE', #23470 ) ;
#22691=FACE_OUTER_BOUND ( 'NONE', #9041, .T. ) ;
#22700=ORIENTED_EDGE ( 'NONE', *, *, #29224, .T. ) ;
#22705=ORIENTED_EDGE ( 'NONE', *, *, #23445, .F. ) ;
#22725=DIRECTION ( 'NONE',  ( 0.000000000000000000, -1.000000000000000000, 0.000000000000000000 ) ) ;
#22732=VECTOR ( 'NONE', #8324, 1000.000000000000000 ) ;
#22741=VERTEX_POINT ( 'NONE', #9907 ) ;
#22743=CARTESIAN_POINT ( 'NONE',  ( 49.66189766834159514, 69.99759634488681570, 19.83556485701890892 ) ) ;
#22745=ADVANCED_FACE ( 'NONE', ( #21908 ), #19111, .T. ) ;
#22747=ORIENTED_EDGE ( 'NONE', *, *, #12967, .T. ) ;
#22756=CARTESIAN_POINT ( 'NONE',  ( -40.00000000000002842, 90.00000000000001421, 27.49999999999983658 ) ) ;
#22791=AXIS2_PLACEMENT_3D ( 'NONE', #13765, #4099, #23262 ) ;
#22797=CIRCLE ( 'NONE', #11845, 6.999999999999999112 ) ;
#22811=CIRCLE ( 'NONE', #15344, 34.99999999999933920 ) ;
#22825=FACE_OUTER_BOUND ( 'NONE', #14960, .T. ) ;
#22848=DIRECTION ( 'NONE',  ( 0.000000000000000000, 1.000000000000000000, -0.000000000000000000 ) ) ;
#22856=FACE_BOUND ( 'NONE', #27049, .T. ) ;
#22872=ORIENTED_EDGE ( 'NONE', *, *, #26147, .F. ) ;
#22879=ORIENTED_EDGE ( 'NONE', *, *, #10806, .T. ) ;
#22881=ORIENTED_EDGE ( 'NONE', *, *, #18979, .F. ) ;
#22896=CIRCLE ( 'NONE', #12963, 50.00000000000000000 ) ;
#22901=CARTESIAN_POINT ( 'NONE',  ( 48.02684528033974942, 69.90336711249833002, 16.52639074396786611 ) ) ;
#22904=VERTEX_POINT ( 'NONE', #10795 ) ;
#22910=EDGE_CURVE ( 'NONE', #5078, #20897, #15465, .T. ) ;
#22948=EDGE_CURVE ( 'NONE', #2627, #24377, #11561, .T. ) ;
#22970=CYLINDRICAL_SURFACE ( 'NONE', #5834, 10.00000000000000178 ) ;
#22975=ORIENTED_EDGE ( 'NONE', *, *, #17536, .F. ) ;
#22981=ORIENTED_EDGE ( 'NONE', *, *, #13785, .T. ) ;
#22985=EDGE_LOOP ( 'NONE', ( #11787, #7386 ) ) ;
#22986=CIRCLE ( 'NONE', #9541, 6.999999999999999112 ) ;
#22989=ORIENTED_EDGE ( 'NONE', *, *, #7646, .T. ) ;
#22997=CARTESIAN_POINT ( 'NONE',  ( 39.99999999999998579, 70.00000000000000000, 12.49999999999999112 ) ) ;
#23005=FACE_OUTER_BOUND ( 'NONE', #30457, .T. ) ;
#23006=EDGE_CURVE ( 'NONE', #9226, #25866, #1736, .T. ) ;
#23008=ORIENTED_EDGE ( 'NONE', *, *, #482, .F. ) ;
#23009=FACE_BOUND ( 'NONE', #25088, .T. ) ;
#23026=CIRCLE ( 'NONE', #3118, 17.00000000000000000 ) ;
#23029=ORIENTED_EDGE ( 'NONE', *, *, #25180, .T. ) ;
#23045=CIRCLE ( 'NONE', #634, 7.500000000000013323 ) ;
#23046=CARTESIAN_POINT ( 'NONE',  ( -38.00000000000000711, 80.00000000000000000, 17.91742430504400119 ) ) ;
#23073=DIRECTION ( 'NONE',  ( -0.000000000000000000, 1.000000000000000000, -0.000000000000000000 ) ) ;
#23078=ORIENTED_EDGE ( 'NONE', *, *, #3472, .F. ) ;
#23079=CARTESIAN_POINT ( 'NONE',  ( -40.00000000000002842, 80.00000000000001421, 57.50000000000015632 ) ) ;
#23088=DIRECTION ( 'NONE',  ( -1.000000000000000000, 0.000000000000000000, 0.000000000000000000 ) ) ;
#23090=CARTESIAN_POINT ( 'NONE',  ( 37.16608720827707657, 36.86186943028246787, 12.49999999999999112 ) ) ;
#23091=EDGE_CURVE ( 'NONE', #22640, #9013, #9990, .T. ) ;
#23092=VECTOR ( 'NONE', #3427, 1000.000000000000000 ) ;
#23093=ORIENTED_EDGE ( 'NONE', *, *, #15085, .T. ) ;
#23104=ORIENTED_EDGE ( 'NONE', *, *, #6085, .F. ) ;
#23109=AXIS2_PLACEMENT_3D ( 'NONE', #14153, #16660, #11671 ) ;
#23123=EDGE_CURVE ( 'NONE', #30496, #3050, #17777, .T. ) ;
#23126=CARTESIAN_POINT ( 'NONE',  ( -50.00000000000000000, -50.00000000000000000, 12.49999999999999112 ) ) ;
#23131=EDGE_CURVE ( 'NONE', #9013, #19648, #26670, .T. ) ;
#23132=CARTESIAN_POINT ( 'NONE',  ( -40.00000000000002842, 80.00000000000001421, 17.49999999999982947 ) ) ;
#23150=DIRECTION ( 'NONE',  ( 0.000000000000000000, 0.000000000000000000, 1.000000000000000000 ) ) ;
#23151=CARTESIAN_POINT ( 'NONE',  ( -46.43819574214524692, 69.68628862962340520, 14.81935245954445435 ) ) ;
#23155=DIRECTION ( 'NONE',  ( -0.000000000000000000, 0.000000000000000000, 1.000000000000000000 ) ) ;
#23167=CARTESIAN_POINT ( 'NONE',  ( 37.16608720827707657, 65.00000000000000000, 50.49999999999998579 ) ) ;
#23203=CARTESIAN_POINT ( 'NONE',  ( -40.00000000000000000, 90.00000000000001421, 22.49999999999999289 ) ) ;
#23213=AXIS2_PLACEMENT_3D ( 'NONE', #7676, #26696, #5327 ) ;
#23250=DIRECTION ( 'NONE',  ( 1.000000000000000000, 0.000000000000000000, 0.000000000000000000 ) ) ;
#23257=DIRECTION ( 'NONE',  ( 0.000000000000000000, 0.000000000000000000, 1.000000000000000000 ) ) ;
#23259=PLANE ( 'NONE',  #5601 ) ;
#23262=DIRECTION ( 'NONE',  ( 0.000000000000000000, 0.000000000000000000, 1.000000000000000000 ) ) ;
#23295=ADVANCED_FACE ( 'NONE', ( #15584, #20712 ), #13714, .T. ) ;
#23300=CIRCLE ( 'NONE', #8873, 53.00000000000000711 ) ;
#23313=CARTESIAN_POINT ( 'NONE',  ( -43.31339426922971114, 68.85174796075946801, 13.05946217696219236 ) ) ;
#23321=FACE_OUTER_BOUND ( 'NONE', #7756, .T. ) ;
#23327=CARTESIAN_POINT ( 'NONE',  ( -44.99999999999955236, -4.926614671774132148E-13, 57.49999999999999289 ) ) ;
#23338=CARTESIAN_POINT ( 'NONE',  ( 4.510281037539698445E-13, -4.926614671774132148E-13, 62.49999999999999289 ) ) ;
#23339=EDGE_CURVE ( 'NONE', #19467, #19119, #15427, .T. ) ;
#23341=ORIENTED_EDGE ( 'NONE', *, *, #232, .F. ) ;
#23342=CYLINDRICAL_SURFACE ( 'NONE', #8885, 15.00000000000000000 ) ;
#23363=CARTESIAN_POINT ( 'NONE',  ( -49.48635302761310584, 69.99362080440305078, 55.68038323789210864 ) ) ;
#23407=VERTEX_POINT ( 'NONE', #7464 ) ;
#23409=VERTEX_POINT ( 'NONE', #23512 ) ;
#23412=DIRECTION ( 'NONE',  ( 0.000000000000000000, 0.000000000000000000, 1.000000000000000000 ) ) ;
#23413=EDGE_LOOP ( 'NONE', ( #9090, #16410, #5620, #13210 ) ) ;
#23419=CARTESIAN_POINT ( 'NONE',  ( 50.00000000000045475, -4.865382331816764069E-13, 65.49999999999998579 ) ) ;
#23435=ORIENTED_EDGE ( 'NONE', *, *, #436, .F. ) ;
#23436=VECTOR ( 'NONE', #25534, 1000.000000000000000 ) ;
#23445=EDGE_CURVE ( 'NONE', #12801, #19418, #19922, .T. ) ;
#23450=DIRECTION ( 'NONE',  ( 1.000000000000000000, 0.000000000000000000, 0.000000000000000000 ) ) ;
#23465=DIRECTION ( 'NONE',  ( 0.000000000000000000, 1.000000000000000000, -0.000000000000000000 ) ) ;
#23468=CARTESIAN_POINT ( 'NONE',  ( 37.16608720827707657, 65.00000000000000000, 97.07879600563551037 ) ) ;
#23470=CARTESIAN_POINT ( 'NONE',  ( -37.16608720827707657, 65.00000000000000000, 50.49999999999998579 ) ) ;
#23472=VERTEX_POINT ( 'NONE', #1933 ) ;
#23485=DIRECTION ( 'NONE',  ( -1.000000000000000000, 0.000000000000000000, 0.000000000000000000 ) ) ;
#23512=CARTESIAN_POINT ( 'NONE',  ( 66.99999999999998579, -50.00000000000000000, 62.49999999999999289 ) ) ;
#23516=CARTESIAN_POINT ( 'NONE',  ( 39.99999999999998579, 80.00000000000001421, 22.49999999999999289 ) ) ;
#23524=CYLINDRICAL_SURFACE ( 'NONE', #1132, 5.000000000000004441 ) ;
#23525=FACE_OUTER_BOUND ( 'NONE', #15726, .T. ) ;
#23537=VERTEX_POINT ( 'NONE', #13502 ) ;
#23551=AXIS2_PLACEMENT_3D ( 'NONE', #30518, #13850, #5212 ) ;
#23552=ORIENTED_EDGE ( 'NONE', *, *, #17188, .F. ) ;
#23554=CIRCLE ( 'NONE', #25064, 7.500000000000000000 ) ;
#23565=DIRECTION ( 'NONE',  ( 0.000000000000000000, 0.000000000000000000, -1.000000000000000000 ) ) ;
#23576=VECTOR ( 'NONE', #3742, 1000.000000000000000 ) ;
#23634=ORIENTED_EDGE ( 'NONE', *, *, #7446, .F. ) ;
#23662=DIRECTION ( 'NONE',  ( 0.000000000000000000, 0.000000000000000000, 1.000000000000000000 ) ) ;
#23666=EDGE_LOOP ( 'NONE', ( #10276, #16463, #16135, #2620, #16243, #23435, #11692 ) ) ;
#23670=ORIENTED_EDGE ( 'NONE', *, *, #28125, .T. ) ;
#23671=EDGE_CURVE ( 'NONE', #346, #119, #21412, .T. ) ;
#23672=DIRECTION ( 'NONE',  ( 0.000000000000000000, 0.000000000000000000, 1.000000000000000000 ) ) ;
#23673=CARTESIAN_POINT ( 'NONE',  ( 52.16608720827707657, 51.86186943028246787, 57.49999999999999289 ) ) ;
#23674=AXIS2_PLACEMENT_3D ( 'NONE', #16775, #28339, #21295 ) ;
#23678=ORIENTED_EDGE ( 'NONE', *, *, #29975, .F. ) ;
#23685=VERTEX_POINT ( 'NONE', #196 ) ;
#23691=AXIS2_PLACEMENT_3D ( 'NONE', #9120, #28147, #18186 ) ;
#23692=LINE ( 'NONE', #21511, #4433 ) ;
#23700=ORIENTED_EDGE ( 'NONE', *, *, #9947, .T. ) ;
#23701=AXIS2_PLACEMENT_3D ( 'NONE', #11853, #4822, #23847 ) ;
#23702=LINE ( 'NONE', #6879, #28238 ) ;
#23716=AXIS2_PLACEMENT_3D ( 'NONE', #15648, #13168, #3507 ) ;
#23737=ORIENTED_EDGE ( 'NONE', *, *, #3486, .T. ) ;
#23744=ORIENTED_EDGE ( 'NONE', *, *, #4928, .T. ) ;
#23745=CARTESIAN_POINT ( 'NONE',  ( 46.99999999999998579, 87.00000000000001421, 0.000000000000000000 ) ) ;
#23750=AXIS2_PLACEMENT_3D ( 'NONE', #9582, #4445, #23450 ) ;
#23758=PLANE ( 'NONE',  #25577 ) ;
#23759=AXIS2_PLACEMENT_3D ( 'NONE', #20683, #11037, #6043 ) ;
#23762=CIRCLE ( 'NONE', #11823, 7.500000000000000000 ) ;
#23763=CARTESIAN_POINT ( 'NONE',  ( 39.99999999999998579, 90.00000000000001421, 22.49999999999999289 ) ) ;
#23767=CARTESIAN_POINT ( 'NONE',  ( 42.49999999999998579, -50.00000000000000000, 12.49999999999999112 ) ) ;
#23785=CIRCLE ( 'NONE', #10357, 3.000000000000002665 ) ;
#23823=ORIENTED_EDGE ( 'NONE', *, *, #27648, .T. ) ;
#23833=EDGE_CURVE ( 'NONE', #8898, #22640, #15470, .T. ) ;
#23840=CIRCLE ( 'NONE', #17380, 15.00000000000000000 ) ;
#23847=DIRECTION ( 'NONE',  ( -1.000000000000000000, 0.000000000000000000, 0.000000000000000000 ) ) ;
#23863=VERTEX_POINT ( 'NONE', #8161 ) ;
#23876=LINE ( 'NONE', #21524, #22480 ) ;
#23881=CYLINDRICAL_SURFACE ( 'NONE', #20743, 3.000000000000002665 ) ;
#23905=VERTEX_POINT ( 'NONE', #25463 ) ;
#23923=CYLINDRICAL_SURFACE ( 'NONE', #17107, 7.500000000000013323 ) ;
#23936=EDGE_LOOP ( 'NONE', ( #14340, #22700, #12891, #26909 ) ) ;
#23938=DIRECTION ( 'NONE',  ( 0.000000000000000000, 0.000000000000000000, -1.000000000000000000 ) ) ;
#23944=ORIENTED_EDGE ( 'NONE', *, *, #14699, .T. ) ;
#23955=EDGE_LOOP ( 'NONE', ( #1588, #8124, #13224, #16498 ) ) ;
#23968=CARTESIAN_POINT ( 'NONE',  ( -48.17766558237416064, 69.91760311152096108, 58.26458773037651895 ) ) ;
#24000=CARTESIAN_POINT ( 'NONE',  ( 69.99999999999998579, -50.00000000000000000, 12.49999999999999112 ) ) ;
#24027=EDGE_CURVE ( 'NONE', #977, #10854, #29901, .T. ) ;
#24053=VERTEX_POINT ( 'NONE', #17155 ) ;
#24060=DIRECTION ( 'NONE',  ( -1.000000000000000000, 0.000000000000000000, 0.000000000000000000 ) ) ;
#24081=FACE_OUTER_BOUND ( 'NONE', #24097, .T. ) ;
#24091=DIRECTION ( 'NONE',  ( 0.000000000000000000, -0.000000000000000000, -1.000000000000000000 ) ) ;
#24097=EDGE_LOOP ( 'NONE', ( #12371, #25996, #12714, #8816 ) ) ;
#24102=DIRECTION ( 'NONE',  ( -0.000000000000000000, -0.000000000000000000, -1.000000000000000000 ) ) ;
#24106=CARTESIAN_POINT ( 'NONE',  ( -65.00000000000000000, -36.86186943028246787, 12.49999999999999112 ) ) ;
#24109=LINE ( 'NONE', #16945, #13318 ) ;
#24110=DIRECTION ( 'NONE',  ( 1.000000000000000000, -0.000000000000000000, 0.000000000000000000 ) ) ;
#24111=LINE ( 'NONE', #16790, #20267 ) ;
#24114=DIRECTION ( 'NONE',  ( -0.000000000000000000, -0.000000000000000000, -1.000000000000000000 ) ) ;
#24124=LINE ( 'NONE', #14767, #15362 ) ;
#24126=CARTESIAN_POINT ( 'NONE',  ( -50.00000000000000000, -67.00000000000000000, 62.49999999999999289 ) ) ;
#24140=LINE ( 'NONE', #17128, #26036 ) ;
#24142=CARTESIAN_POINT ( 'NONE',  ( 49.99999999999998579, 87.00000000000001421, 22.49999999999999289 ) ) ;
#24152=VERTEX_POINT ( 'NONE', #18897 ) ;
#24182=FACE_OUTER_BOUND ( 'NONE', #30613, .T. ) ;
#24189=LINE ( 'NONE', #2842, #29777 ) ;
#24193=AXIS2_PLACEMENT_3D ( 'NONE', #18574, #21501, #2179 ) ;
#24197=ORIENTED_EDGE ( 'NONE', *, *, #436, .T. ) ;
#24213=LINE ( 'NONE', #14864, #3327 ) ;
#24236=VERTEX_POINT ( 'NONE', #22756 ) ;
#24239=DIRECTION ( 'NONE',  ( -1.000000000000000000, 0.000000000000000000, 0.000000000000000000 ) ) ;
#24243=DIRECTION ( 'NONE',  ( -0.000000000000000000, 1.000000000000000000, -0.000000000000000000 ) ) ;
#24270=DIRECTION ( 'NONE',  ( 0.000000000000000000, 1.000000000000000000, 0.000000000000000000 ) ) ;
#24320=LINE ( 'NONE', #17143, #16318 ) ;
#24356=CARTESIAN_POINT ( 'NONE',  ( -46.04937532021984481, 69.44700638503979917, 60.46533948008040937 ) ) ;
#24365=ORIENTED_EDGE ( 'NONE', *, *, #210, .T. ) ;
#24377=VERTEX_POINT ( 'NONE', #16509 ) ;
#24385=DIRECTION ( 'NONE',  ( 0.000000000000000000, 1.000000000000000000, 0.000000000000000000 ) ) ;
#24392=CARTESIAN_POINT ( 'NONE',  ( -37.16608720827707657, -51.86186943028246787, 12.49999999999999112 ) ) ;
#24397=EDGE_LOOP ( 'NONE', ( #20720, #27108, #4018, #21414 ) ) ;
#24401=DIRECTION ( 'NONE',  ( -0.000000000000000000, -0.000000000000000000, 1.000000000000000000 ) ) ;
#24406=DIRECTION ( 'NONE',  ( 0.000000000000000000, 0.000000000000000000, -1.000000000000000000 ) ) ;
#24422=EDGE_CURVE ( 'NONE', #9325, #9621, #9493, .T. ) ;
#24426=B_SPLINE_CURVE_WITH_KNOTS ( 'NONE', 3,
 ( #15528, #25044, #26939, #15059, #24573, #25818, #11474, #20663, #11167, #20817, #1653, #13811, #27999, #23151, #30036, #15994, #25662, #23313, #18035, #8821, #13359, #4282, #8980, #30629 ),
 .UNSPECIFIED., .F., .F.,
 ( 4, 2, 2, 2, 2, 2, 2, 2, 2, 2, 2, 4 ),
 ( 0.000000000000000000, 0.002009081642066640975, 0.003013622463099961679, 0.004018163284133281950, 0.006027244926199938971, 0.007031785747233264446, 0.008036326568266588186, 0.01004540821033321832, 0.01205448985239984845, 0.01305903067343317826, 0.01406357149446650807, 0.01607265313653316596 ),
 .UNSPECIFIED. ) ;
#24435=ORIENTED_EDGE ( 'NONE', *, *, #19707, .T. ) ;
#24451=EDGE_LOOP ( 'NONE', ( #13751, #25164, #15935, #4962 ) ) ;
#24475=EDGE_CURVE ( 'NONE', #8092, #18, #4506, .T. ) ;
#24480=ORIENTED_EDGE ( 'NONE', *, *, #18563, .T. ) ;
#24483=LINE ( 'NONE', #5469, #7749 ) ;
#24487=EDGE_CURVE ( 'NONE', #20113, #11497, #25919, .T. ) ;
#24493=VERTEX_POINT ( 'NONE', #15394 ) ;
#24496=CARTESIAN_POINT ( 'NONE',  ( 57.49999999999998579, -50.00000000000000000, 62.49999999999999289 ) ) ;
#24501=ORIENTED_EDGE ( 'NONE', *, *, #26177, .T. ) ;
#24514=CARTESIAN_POINT ( 'NONE',  ( -64.99999999999998579, 36.86186943028246787, 57.49999999999999289 ) ) ;
#24524=CIRCLE ( 'NONE', #11092, 3.000000000000002665 ) ;
#24535=DIRECTION ( 'NONE',  ( 1.000000000000000000, 0.000000000000000000, 4.565061778886335400E-17 ) ) ;
#24542=VECTOR ( 'NONE', #13399, 1000.000000000000000 ) ;
#24560=DIRECTION ( 'NONE',  ( 0.000000000000000000, 1.000000000000000000, 0.000000000000000000 ) ) ;
#24568=CARTESIAN_POINT ( 'NONE',  ( -4.163336342344337027E-14, 1.387778780781445676E-14, 92.49999999999998579 ) ) ;
#24571=FACE_OUTER_BOUND ( 'NONE', #8108, .T. ) ;
#24573=CARTESIAN_POINT ( 'NONE',  ( -49.64645017045302922, 69.99712838247133107, 19.84290309017789866 ) ) ;
#24579=DIRECTION ( 'NONE',  ( 1.224646799147353207E-16, 1.000000000000000000, -0.000000000000000000 ) ) ;
#24598=FACE_BOUND ( 'NONE', #27563, .T. ) ;
#24603=ADVANCED_FACE ( 'NONE', ( #24598, #3556, #13078, #22568, #26811, #1221 ), #14780, .T. ) ;
#24609=DIRECTION ( 'NONE',  ( 0.000000000000000000, -1.000000000000000000, 0.000000000000000000 ) ) ;
#24610=CARTESIAN_POINT ( 'NONE',  ( 45.00000000000045475, -4.871505565812501079E-13, 82.49999999999998579 ) ) ;
#24618=ORIENTED_EDGE ( 'NONE', *, *, #18064, .F. ) ;
#24637=EDGE_CURVE ( 'NONE', #16462, #7391, #30370, .T. ) ;
#24646=ORIENTED_EDGE ( 'NONE', *, *, #24027, .F. ) ;
#24659=CARTESIAN_POINT ( 'NONE',  ( 41.02680411063263932, 65.11861831110995524, 62.46341751033051537 ) ) ;
#24670=VERTEX_POINT ( 'NONE', #18520 ) ;
#24673=CARTESIAN_POINT ( 'NONE',  ( 49.99999999999998579, 70.00000000000000000, 52.49999999999999289 ) ) ;
#24686=DIRECTION ( 'NONE',  ( 0.000000000000000000, 0.000000000000000000, -1.000000000000000000 ) ) ;
#24707=ORIENTED_EDGE ( 'NONE', *, *, #18336, .T. ) ;
#24720=AXIS2_PLACEMENT_3D ( 'NONE', #23745, #3862, #28302 ) ;
#24740=ORIENTED_EDGE ( 'NONE', *, *, #8260, .F. ) ;
#24742=LINE ( 'NONE', #20380, #29888 ) ;
#24751=FACE_OUTER_BOUND ( 'NONE', #14422, .T. ) ;
#24754=ORIENTED_EDGE ( 'NONE', *, *, #17361, .T. ) ;
#24756=EDGE_LOOP ( 'NONE', ( #27581, #1257 ) ) ;
#24758=AXIS2_PLACEMENT_3D ( 'NONE', #28105, #26059, #6726 ) ;
#24760=AXIS2_PLACEMENT_3D ( 'NONE', #6589, #29850, #30442 ) ;
#24762=CARTESIAN_POINT ( 'NONE',  ( 42.49999999999998579, 50.00000000000000000, 62.49999999999999289 ) ) ;
#24771=ORIENTED_EDGE ( 'NONE', *, *, #30132, .F. ) ;
#24773=PRODUCT_DEFINITION ( 'UNKNOWN', '', #13892, #15745 ) ;
#24790=CYLINDRICAL_SURFACE ( 'NONE', #29607, 29.99999999999928946 ) ;
#24794=DIRECTION ( 'NONE',  ( -0.000000000000000000, -0.000000000000000000, 1.000000000000000000 ) ) ;
#24800=CARTESIAN_POINT ( 'NONE',  ( 0.000000000000000000, 75.00000000000001421, 50.49999999999998579 ) ) ;
#24806=AXIS2_PLACEMENT_3D ( 'NONE', #7200, #23565, #28570 ) ;
#24813=AXIS2_PLACEMENT_3D ( 'NONE', #16140, #22848, #25348 ) ;
#24822=CARTESIAN_POINT ( 'NONE',  ( 44.60412398304908521, 68.57966167107747424, 61.38406682071050824 ) ) ;
#24827=CARTESIAN_POINT ( 'NONE',  ( -65.00000000000000000, -70.00000000000000000, 57.49999999999999289 ) ) ;
#24832=AXIS2_PLACEMENT_3D ( 'NONE', #2869, #12393, #21893 ) ;
#24839=EDGE_LOOP ( 'NONE', ( #27467, #29329, #3630, #19417, #10492, #23678 ) ) ;
#24855=AXIS2_PLACEMENT_3D ( 'NONE', #17069, #2731, #380 ) ;
#24873=ORIENTED_EDGE ( 'NONE', *, *, #16994, .F. ) ;
#24882=EDGE_LOOP ( 'NONE', ( #16214, #23700, #13737, #2707, #7976, #6090 ) ) ;
#24889=ADVANCED_FACE ( 'NONE', ( #19624 ), #5286, .F. ) ;
#24901=ORIENTED_EDGE ( 'NONE', *, *, #16788, .F. ) ;
#24907=DIRECTION ( 'NONE',  ( -1.000000000000000000, 0.000000000000000000, 0.000000000000000000 ) ) ;
#24919=ORIENTED_EDGE ( 'NONE', *, *, #238, .T. ) ;
#24923=AXIS2_PLACEMENT_3D ( 'NONE', #11566, #27806, #21055 ) ;
#24926=CARTESIAN_POINT ( 'NONE',  ( 49.99999999999998579, -50.00000000000000000, 12.49999999999999112 ) ) ;
#24935=CARTESIAN_POINT ( 'NONE',  ( 49.99999999999998579, 50.00000000000000000, 97.07879600563551037 ) ) ;
#24938=ORIENTED_EDGE ( 'NONE', *, *, #10523, .F. ) ;
#24941=CARTESIAN_POINT ( 'NONE',  ( 4.510281037539698445E-13, -4.926614671774132148E-13, 77.49999999999998579 ) ) ;
#24944=CARTESIAN_POINT ( 'NONE',  ( -70.00000000000000000, 50.00000000000000000, 59.49999999999999289 ) ) ;
#24948=VERTEX_POINT ( 'NONE', #21969 ) ;
#24953=DIRECTION ( 'NONE',  ( 0.000000000000000000, -1.000000000000000000, 0.000000000000000000 ) ) ;
#24956=FACE_OUTER_BOUND ( 'NONE', #17906, .T. ) ;
#24958=EDGE_LOOP ( 'NONE', ( #5343, #218, #29881, #23008 ) ) ;
#24972=CARTESIAN_POINT ( 'NONE',  ( 45.56537712369228643, 69.19660825136207905, 60.81054171467580716 ) ) ;
#24984=CIRCLE ( 'NONE', #25489, 3.000000000000002665 ) ;
#25003=CARTESIAN_POINT ( 'NONE',  ( -4.163336342344337027E-14, 1.387778780781445676E-14, 67.49999999999997158 ) ) ;
#25018=ORIENTED_EDGE ( 'NONE', *, *, #18101, .F. ) ;
#25019=DIRECTION ( 'NONE',  ( -0.000000000000000000, 1.000000000000000000, -0.000000000000000000 ) ) ;
#25029=DIRECTION ( 'NONE',  ( -0.000000000000000000, -0.000000000000000000, 1.000000000000000000 ) ) ;
#25044=CARTESIAN_POINT ( 'NONE',  ( -50.00000000000001421, 70.00000000000001421, 21.82070599434954161 ) ) ;
#25063=VERTEX_POINT ( 'NONE', #26469 ) ;
#25064=AXIS2_PLACEMENT_3D ( 'NONE', #1479, #20490, #1157 ) ;
#25080=CARTESIAN_POINT ( 'NONE',  ( 66.99999999999998579, 50.00000000000000000, 62.49999999999999289 ) ) ;
#25088=EDGE_LOOP ( 'NONE', ( #7230, #30550 ) ) ;
#25093=EDGE_LOOP ( 'NONE', ( #23634, #6217, #8591, #7249 ) ) ;
#25095=CARTESIAN_POINT ( 'NONE',  ( -70.00000000000000000, -50.00000000000000000, 59.49999999999999289 ) ) ;
#25099=CARTESIAN_POINT ( 'NONE',  ( -42.49999999999998579, 50.00000000000000000, 97.07879600563551037 ) ) ;
#25101=EDGE_CURVE ( 'NONE', #15798, #498, #5102, .T. ) ;
#25109=LINE ( 'NONE', #24800, #26275 ) ;
#25117=DIRECTION ( 'NONE',  ( -0.000000000000000000, -1.000000000000000000, -0.000000000000000000 ) ) ;
#25135=DIRECTION ( 'NONE',  ( 0.000000000000000000, -0.000000000000000000, 1.000000000000000000 ) ) ;
#25164=ORIENTED_EDGE ( 'NONE', *, *, #14903, .T. ) ;
#25178=VERTEX_POINT ( 'NONE', #5563 ) ;
#25180=EDGE_CURVE ( 'NONE', #12762, #2167, #11530, .T. ) ;
#25182=DIRECTION ( 'NONE',  ( 0.000000000000000000, 1.000000000000000000, 0.000000000000000000 ) ) ;
#25196=EDGE_CURVE ( 'NONE', #16566, #11965, #15531, .T. ) ;
#25203=VERTEX_POINT ( 'NONE', #1043 ) ;
#25208=EDGE_LOOP ( 'NONE', ( #25482, #9693, #18999, #2162, #4010, #17826 ) ) ;
#25214=ORIENTED_EDGE ( 'NONE', *, *, #12452, .T. ) ;
#25229=AXIS2_PLACEMENT_3D ( 'NONE', #22508, #1008, #15177 ) ;
#25230=CARTESIAN_POINT ( 'NONE',  ( -40.00000000000002842, 80.00000000000001421, 17.49999999999982947 ) ) ;
#25244=ORIENTED_EDGE ( 'NONE', *, *, #9548, .T. ) ;
#25247=CARTESIAN_POINT ( 'NONE',  ( 45.89490515299661411, 69.57600767808649778, 14.41534730701735256 ) ) ;
#25281=LINE ( 'NONE', #6095, #28694 ) ;
#25284=CARTESIAN_POINT ( 'NONE',  ( 39.99999999999998579, 90.00000000000001421, 52.49999999999999289 ) ) ;
#25288=AXIS2_PLACEMENT_3D ( 'NONE', #17558, #8056, #19736 ) ;
#25289=DIRECTION ( 'NONE',  ( 1.000000000000000000, 0.000000000000000000, -0.000000000000000000 ) ) ;
#25307=AXIS2_PLACEMENT_3D ( 'NONE', #30372, #4017, #11040 ) ;
#25314=DIRECTION ( 'NONE',  ( 0.000000000000000000, 0.000000000000000000, -1.000000000000000000 ) ) ;
#25328=VECTOR ( 'NONE', #6764, 1000.000000000000000 ) ;
#25330=APPLICATION_CONTEXT ( 'automotive_design' ) ;
#25331=LINE ( 'NONE', #18162, #26859 ) ;
#25335=ORIENTED_EDGE ( 'NONE', *, *, #20958, .F. ) ;
#25339=ORIENTED_EDGE ( 'NONE', *, *, #30184, .F. ) ;
#25348=DIRECTION ( 'NONE',  ( 0.000000000000000000, 0.000000000000000000, -1.000000000000000000 ) ) ;
#25354=CARTESIAN_POINT ( 'NONE',  ( -37.16608720827707657, 65.00000000000000000, 15.49999999999998579 ) ) ;
#25355=FACE_OUTER_BOUND ( 'NONE', #18987, .T. ) ;
#25360=CARTESIAN_POINT ( 'NONE',  ( 53.00000000000045475, -4.861708391419322267E-13, 62.49999999999998579 ) ) ;
#25361=DIRECTION ( 'NONE',  ( -1.000000000000000000, 0.000000000000000000, 0.000000000000000000 ) ) ;
#25362=DIRECTION ( 'NONE',  ( 1.000000000000000000, 0.000000000000000000, 0.000000000000000000 ) ) ;
#25371=FACE_BOUND ( 'NONE', #21941, .T. ) ;
#25376=VECTOR ( 'NONE', #2037, 1000.000000000000000 ) ;
#25398=CARTESIAN_POINT ( 'NONE',  ( 57.49999999999998579, 50.00000000000000000, 97.07879600563551037 ) ) ;
#25413=EDGE_CURVE ( 'NONE', #498, #11642, #9528, .T. ) ;
#25421=DIRECTION ( 'NONE',  ( 1.000000000000000000, 0.000000000000000000, 0.000000000000000000 ) ) ;
#25424=ORIENTED_EDGE ( 'NONE', *, *, #3097, .F. ) ;
#25427=EDGE_LOOP ( 'NONE', ( #15864, #9875 ) ) ;
#25428=DIRECTION ( 'NONE',  ( 0.000000000000000000, 0.000000000000000000, 1.000000000000000000 ) ) ;
#25429=EDGE_CURVE ( 'NONE', #24493, #3904, #30797, .T. ) ;
#25437=ORIENTED_EDGE ( 'NONE', *, *, #29414, .T. ) ;
#25445=AXIS2_PLACEMENT_3D ( 'NONE', #16969, #6999, #26487 ) ;
#25448=VERTEX_POINT ( 'NONE', #28321 ) ;
#25463=CARTESIAN_POINT ( 'NONE',  ( -40.00000000000002842, 90.00000000000001421, 57.50000000000015632 ) ) ;
#25479=LINE ( 'NONE', #18300, #28767 ) ;
#25482=ORIENTED_EDGE ( 'NONE', *, *, #25101, .F. ) ;
#25485=VERTEX_POINT ( 'NONE', #16456 ) ;
#25487=DIRECTION ( 'NONE',  ( 0.000000000000000000, 1.000000000000000000, 0.000000000000000000 ) ) ;
#25489=AXIS2_PLACEMENT_3D ( 'NONE', #3953, #13474, #23412 ) ;
#25514=DIRECTION ( 'NONE',  ( 0.000000000000000000, 1.000000000000000000, 0.000000000000000000 ) ) ;
#25524=VERTEX_POINT ( 'NONE', #3635 ) ;
#25534=DIRECTION ( 'NONE',  ( -0.000000000000000000, 1.000000000000000000, -0.000000000000000000 ) ) ;
#25543=ORIENTED_EDGE ( 'NONE', *, *, #10503, .F. ) ;
#25556=AXIS2_PLACEMENT_3D ( 'NONE', #27896, #6519, #9890 ) ;
#25562=ORIENTED_EDGE ( 'NONE', *, *, #9968, .F. ) ;
#25577=AXIS2_PLACEMENT_3D ( 'NONE', #16747, #26263, #12084 ) ;
#25582=AXIS2_PLACEMENT_3D ( 'NONE', #29626, #8112, #756 ) ;
#25598=CARTESIAN_POINT ( 'NONE',  ( -4.163336342344337027E-14, 1.387778780781445676E-14, 77.49999999999998579 ) ) ;
#25599=EDGE_CURVE ( 'NONE', #4862, #12729, #24984, .T. ) ;
#25609=ORIENTED_EDGE ( 'NONE', *, *, #14117, .F. ) ;
#25617=CARTESIAN_POINT ( 'NONE',  ( -70.00000000000000000, 50.00000000000000000, 12.49999999999999112 ) ) ;
#25625=FACE_OUTER_BOUND ( 'NONE', #26960, .T. ) ;
#25628=DIRECTION ( 'NONE',  ( 0.000000000000000000, -1.000000000000000000, 0.000000000000000000 ) ) ;
#25632=EDGE_CURVE ( 'NONE', #12729, #14399, #23876, .T. ) ;
#25633=CARTESIAN_POINT ( 'NONE',  ( -40.00000000000002842, 90.00000000000001421, 47.50000000000014921 ) ) ;
#25637=DIRECTION ( 'NONE',  ( 0.000000000000000000, 0.000000000000000000, 1.000000000000000000 ) ) ;
#25651=DIRECTION ( 'NONE',  ( 0.000000000000000000, 0.000000000000000000, -1.000000000000000000 ) ) ;
#25662=CARTESIAN_POINT ( 'NONE',  ( -44.20831430623121605, 69.15340090750629543, 13.40607705188479670 ) ) ;
#25667=CARTESIAN_POINT ( 'NONE',  ( -47.00000000000000000, 90.00000000000001421, 52.49999999999999289 ) ) ;
#25693=CARTESIAN_POINT ( 'NONE',  ( -49.99999999999955236, -4.926614671774132148E-13, 65.49999999999998579 ) ) ;
#25706=VECTOR ( 'NONE', #17427, 1000.000000000000000 ) ;
#25707=CARTESIAN_POINT ( 'NONE',  ( -47.57918908651176793, 69.85400074660304881, 59.03148159615753343 ) ) ;
#25716=ORIENTED_EDGE ( 'NONE', *, *, #12602, .F. ) ;
#25726=DIRECTION ( 'NONE',  ( -0.000000000000000000, 1.000000000000000000, -0.000000000000000000 ) ) ;
#25740=DIRECTION ( 'NONE',  ( 0.000000000000000000, 0.000000000000000000, 1.000000000000000000 ) ) ;
#25758=ORIENTED_EDGE ( 'NONE', *, *, #29583, .F. ) ;
#25762=ORIENTED_EDGE ( 'NONE', *, *, #1572, .F. ) ;
#25790=VERTEX_POINT ( 'NONE', #628 ) ;
#25797=DIRECTION ( 'NONE',  ( -0.000000000000000000, 0.000000000000000000, -1.000000000000000000 ) ) ;
#25806=EDGE_CURVE ( 'NONE', #23863, #15313, #21007, .T. ) ;
#25816=LINE ( 'NONE', #5744, #12647 ) ;
#25818=CARTESIAN_POINT ( 'NONE',  ( -49.44509678728922353, 69.99255420029007269, 19.19783229408952252 ) ) ;
#25826=CARTESIAN_POINT ( 'NONE',  ( 69.99999999999998579, -70.00000000000000000, 12.49999999999999112 ) ) ;
#25854=DIRECTION ( 'NONE',  ( -1.000000000000000000, 0.000000000000000000, 0.000000000000000000 ) ) ;
#25865=ORIENTED_EDGE ( 'NONE', *, *, #14712, .T. ) ;
#25866=VERTEX_POINT ( 'NONE', #29921 ) ;
#25867=CARTESIAN_POINT ( 'NONE',  ( -47.98494098007435582, 69.89927657657921145, 58.52868780040671481 ) ) ;
#25869=TOROIDAL_SURFACE ( 'NONE', #12429, 47.00000000000000000, 3.000000000000000000 ) ;
#25875=VECTOR ( 'NONE', #19263, 1000.000000000000000 ) ;
#25892=DIRECTION ( 'NONE',  ( 1.000000000000000000, 0.000000000000000000, 0.000000000000000000 ) ) ;
#25900=CARTESIAN_POINT ( 'NONE',  ( -70.00000000000000000, 65.00000000000000000, 57.49999999999999289 ) ) ;
#25903=AXIS2_PLACEMENT_3D ( 'NONE', #6495, #14107, #13824 ) ;
#25911=CARTESIAN_POINT ( 'NONE',  ( -50.00000000000000000, 50.00000000000000000, 12.49999999999999112 ) ) ;
#25919=CIRCLE ( 'NONE', #12490, 4.999999999999997335 ) ;
#25950=ORIENTED_EDGE ( 'NONE', *, *, #6576, .F. ) ;
#25963=CARTESIAN_POINT ( 'NONE',  ( -70.00000000000000000, -50.00000000000000000, 12.49999999999999112 ) ) ;
#25966=ORIENTED_EDGE ( 'NONE', *, *, #10765, .F. ) ;
#25989=ORIENTED_EDGE ( 'NONE', *, *, #10545, .F. ) ;
#25996=ORIENTED_EDGE ( 'NONE', *, *, #7480, .T. ) ;
#26001=ORIENTED_EDGE ( 'NONE', *, *, #22555, .T. ) ;
#26011=DIRECTION ( 'NONE',  ( -0.000000000000000000, -0.000000000000000000, 1.000000000000000000 ) ) ;
#26017=EDGE_LOOP ( 'NONE', ( #1295, #9648 ) ) ;
#26019=CARTESIAN_POINT ( 'NONE',  ( -47.36551906495753883, 69.82702131092923992, 59.27138182264830135 ) ) ;
#26036=VECTOR ( 'NONE', #14788, 1000.000000000000000 ) ;
#26039=VERTEX_POINT ( 'NONE', #24106 ) ;
#26050=PLANE ( 'NONE',  #3387 ) ;
#26059=DIRECTION ( 'NONE',  ( 0.000000000000000000, 0.000000000000000000, -1.000000000000000000 ) ) ;
#26081=DIRECTION ( 'NONE',  ( 1.000000000000000000, 0.000000000000000000, 0.000000000000000000 ) ) ;
#26083=CARTESIAN_POINT ( 'NONE',  ( -50.00000000000000000, 70.00000000000000000, 22.49999999999999289 ) ) ;
#26087=CARTESIAN_POINT ( 'NONE',  ( -46.99999999999955236, -4.867219302015485475E-13, 82.49999999999998579 ) ) ;
#26100=EDGE_LOOP ( 'NONE', ( #17359, #1696, #29825, #20189 ) ) ;
#26121=EDGE_LOOP ( 'NONE', ( #6350, #24938, #21450, #25543 ) ) ;
#26147=EDGE_CURVE ( 'NONE', #10252, #9325, #29984, .T. ) ;
#26148=LINE ( 'NONE', #26625, #4811 ) ;
#26155=DIRECTION ( 'NONE',  ( 0.000000000000000000, 0.000000000000000000, -1.000000000000000000 ) ) ;
#26168=VECTOR ( 'NONE', #15781, 1000.000000000000000 ) ;
#26169=DIRECTION ( 'NONE',  ( 0.000000000000000000, 0.000000000000000000, 1.000000000000000000 ) ) ;
#26171=LINE ( 'NONE', #26642, #15264 ) ;
#26177=EDGE_CURVE ( 'NONE', #28625, #12261, #13070, .T. ) ;
#26178=VECTOR ( 'NONE', #11128, 1000.000000000000000 ) ;
#26182=LINE ( 'NONE', #4201, #20076 ) ;
#26208=ORIENTED_EDGE ( 'NONE', *, *, #16053, .T. ) ;
#26225=DIRECTION ( 'NONE',  ( 0.000000000000000000, -0.000000000000000000, -1.000000000000000000 ) ) ;
#26249=ORIENTED_EDGE ( 'NONE', *, *, #23006, .F. ) ;
#26254=CIRCLE ( 'NONE', #11807, 4.999999999999997335 ) ;
#26263=DIRECTION ( 'NONE',  ( 0.000000000000000000, 1.000000000000000000, 0.000000000000000000 ) ) ;
#26264=AXIS2_PLACEMENT_3D ( 'NONE', #25003, #24686, #996 ) ;
#26266=AXIS2_PLACEMENT_3D ( 'NONE', #17960, #8600, #20583 ) ;
#26275=VECTOR ( 'NONE', #945, 1000.000000000000000 ) ;
#26276=VERTEX_POINT ( 'NONE', #27850 ) ;
#26285=VECTOR ( 'NONE', #17602, 1000.000000000000000 ) ;
#26306=DIRECTION ( 'NONE',  ( 0.000000000000000000, 0.000000000000000000, -1.000000000000000000 ) ) ;
#26307=DIRECTION ( 'NONE',  ( 0.000000000000000000, 0.000000000000000000, -1.000000000000000000 ) ) ;
#26318=DIRECTION ( 'NONE',  ( -0.000000000000000000, -0.000000000000000000, 1.000000000000000000 ) ) ;
#26322=CARTESIAN_POINT ( 'NONE',  ( -49.93682080695227654, 70.00028624649445419, 53.79435855004096112 ) ) ;
#26348=ADVANCED_FACE ( 'NONE', ( #26892 ), #1061, .T. ) ;
#26359=ORIENTED_EDGE ( 'NONE', *, *, #11225, .F. ) ;
#26361=DIRECTION ( 'NONE',  ( -0.000000000000000000, -0.000000000000000000, 1.000000000000000000 ) ) ;
#26372=AXIS2_PLACEMENT_3D ( 'NONE', #11381, #20874, #6073 ) ;
#26394=DIRECTION ( 'NONE',  ( 0.000000000000000000, 0.000000000000000000, -1.000000000000000000 ) ) ;
#26399=CARTESIAN_POINT ( 'NONE',  ( -37.16608720827707657, -65.00000000000000000, 12.49999999999999112 ) ) ;
#26400=DIRECTION ( 'NONE',  ( -0.000000000000000000, 1.000000000000000000, 0.000000000000000000 ) ) ;
#26403=CARTESIAN_POINT ( 'NONE',  ( 39.99999999999998579, 80.00000000000001421, 22.49999999999999289 ) ) ;
#26405=CIRCLE ( 'NONE', #19430, 17.00000000000000000 ) ;
#26412=ORIENTED_EDGE ( 'NONE', *, *, #6530, .F. ) ;
#26418=ORIENTED_EDGE ( 'NONE', *, *, #9548, .F. ) ;
#26421=EDGE_LOOP ( 'NONE', ( #7073, #27088, #9110, #5422 ) ) ;
#26430=DIRECTION ( 'NONE',  ( 0.000000000000000000, 0.000000000000000000, -1.000000000000000000 ) ) ;
#26432=CARTESIAN_POINT ( 'NONE',  ( 37.99999999999933920, 0.000000000000000000, 82.49999999999998579 ) ) ;
#26435=CYLINDRICAL_SURFACE ( 'NONE', #11413, 5.000000000000004441 ) ;
#26438=DIRECTION ( 'NONE',  ( -0.000000000000000000, -0.000000000000000000, 1.000000000000000000 ) ) ;
#26439=EDGE_CURVE ( 'NONE', #28591, #7862, #29682, .T. ) ;
#26440=ORIENTED_EDGE ( 'NONE', *, *, #7801, .T. ) ;
#26444=EDGE_CURVE ( 'NONE', #25866, #7224, #22458, .T. ) ;
#26469=CARTESIAN_POINT ( 'NONE',  ( 69.99999999999998579, -50.00000000000000000, 59.49999999999999289 ) ) ;
#26474=EDGE_LOOP ( 'NONE', ( #27512, #17896, #6145, #26923 ) ) ;
#26487=DIRECTION ( 'NONE',  ( -1.000000000000000000, 0.000000000000000000, 0.000000000000000000 ) ) ;
#26505=DIRECTION ( 'NONE',  ( 0.000000000000000000, -0.000000000000000000, 1.000000000000000000 ) ) ;
#26514=AXIS2_PLACEMENT_3D ( 'NONE', #10363, #29233, #2575 ) ;
#26522=ADVANCED_FACE ( 'NONE', ( #25625 ), #23259, .T. ) ;
#26532=ORIENTED_EDGE ( 'NONE', *, *, #17597, .F. ) ;
#26536=VECTOR ( 'NONE', #5876, 1000.000000000000000 ) ;
#26549=DIRECTION ( 'NONE',  ( 1.000000000000000000, 0.000000000000000000, 0.000000000000000000 ) ) ;
#26552=CARTESIAN_POINT ( 'NONE',  ( 39.99999999999998579, 87.00000000000001421, 22.49999999999999289 ) ) ;
#26558=EDGE_CURVE ( 'NONE', #30078, #12825, #9506, .T. ) ;
#26576=ORIENTED_EDGE ( 'NONE', *, *, #2683, .F. ) ;
#26578=EDGE_CURVE ( 'NONE', #19648, #29034, #23, .T. ) ;
#26589=CARTESIAN_POINT ( 'NONE',  ( -2.081668171172168513E-14, 75.00000000000001421, 37.49999999999999289 ) ) ;
#26599=ORIENTED_EDGE ( 'NONE', *, *, #16662, .F. ) ;
#26605=ORIENTED_EDGE ( 'NONE', *, *, #27671, .F. ) ;
#26607=CARTESIAN_POINT ( 'NONE',  ( -38.00000000000000000, 80.00000000000000000, -7.533656238527846826E-15 ) ) ;
#26613=DIRECTION ( 'NONE',  ( -0.000000000000000000, 1.000000000000000000, -0.000000000000000000 ) ) ;
#26625=CARTESIAN_POINT ( 'NONE',  ( -70.00000000000000000, 65.00000000000000000, 12.49999999999999112 ) ) ;
#26642=CARTESIAN_POINT ( 'NONE',  ( -29.99999999999933209, 1.755172820525642916E-14, 67.49999999999997158 ) ) ;
#26649=VERTEX_POINT ( 'NONE', #6735 ) ;
#26666=DIRECTION ( 'NONE',  ( 1.000000000000000000, 0.000000000000000000, 0.000000000000000000 ) ) ;
#26670=LINE ( 'NONE', #3123, #4951 ) ;
#26688=CARTESIAN_POINT ( 'NONE',  ( -67.00000000000000000, 0.000000000000000000, 59.49999999999999289 ) ) ;
#26696=DIRECTION ( 'NONE',  ( 0.000000000000000000, 1.000000000000000000, -0.000000000000000000 ) ) ;
#26723=ORIENTED_EDGE ( 'NONE', *, *, #29756, .F. ) ;
#26745=ADVANCED_FACE ( 'NONE', ( #27158 ), #27010, .T. ) ;
#26765=ADVANCED_FACE ( 'NONE', ( #10464 ), #29497, .T. ) ;
#26766=AXIS2_PLACEMENT_3D ( 'NONE', #27166, #14836, #10472 ) ;
#26777=CARTESIAN_POINT ( 'NONE',  ( -50.00000000000000000, -67.00000000000000000, 59.49999999999999289 ) ) ;
#26782=PLANE ( 'NONE',  #18779 ) ;
#26784=LINE ( 'NONE', #12739, #11789 ) ;
#26792=CARTESIAN_POINT ( 'NONE',  ( 37.99999999999999289, 80.00000000000000000, 15.49999999999998934 ) ) ;
#26793=CIRCLE ( 'NONE', #15750, 15.00000000000000000 ) ;
#26809=DIRECTION ( 'NONE',  ( 0.000000000000000000, 0.000000000000000000, -1.000000000000000000 ) ) ;
#26811=FACE_OUTER_BOUND ( 'NONE', #6016, .T. ) ;
#26813=VECTOR ( 'NONE', #25314, 1000.000000000000000 ) ;
#26833=ORIENTED_EDGE ( 'NONE', *, *, #10750, .F. ) ;
#26845=DIRECTION ( 'NONE',  ( 0.000000000000000000, -1.000000000000000000, 0.000000000000000000 ) ) ;
#26856=CARTESIAN_POINT ( 'NONE',  ( 49.01082926198596823, 69.97703016100948048, 56.88457827394385191 ) ) ;
#26859=VECTOR ( 'NONE', #25019, 1000.000000000000000 ) ;
#26871=CARTESIAN_POINT ( 'NONE',  ( -7.075845757273814415E-16, 65.00000000000000000, 15.49999999999998757 ) ) ;
#26882=ORIENTED_EDGE ( 'NONE', *, *, #18352, .T. ) ;
#26889=EDGE_LOOP ( 'NONE', ( #2479, #10142, #26249, #25424 ) ) ;
#26892=FACE_OUTER_BOUND ( 'NONE', #28778, .T. ) ;
#26901=EDGE_CURVE ( 'NONE', #30435, #10893, #3703, .T. ) ;
#26908=CARTESIAN_POINT ( 'NONE',  ( 49.99999999999998579, -50.00000000000000000, 62.49999999999999289 ) ) ;
#26909=ORIENTED_EDGE ( 'NONE', *, *, #22349, .T. ) ;
#26923=ORIENTED_EDGE ( 'NONE', *, *, #19570, .T. ) ;
#26925=PLANE ( 'NONE',  #10246 ) ;
#26939=CARTESIAN_POINT ( 'NONE',  ( -49.93150111878230035, 70.00033327193624189, 21.15304995801174215 ) ) ;
#26945=ORIENTED_EDGE ( 'NONE', *, *, #10750, .T. ) ;
#26951=ADVANCED_FACE ( 'NONE', ( #27619 ), #20052, .T. ) ;
#26956=ORIENTED_EDGE ( 'NONE', *, *, #14923, .F. ) ;
#26960=EDGE_LOOP ( 'NONE', ( #14307, #16584, #28136, #2708, #27132, #12138 ) ) ;
#26975=CARTESIAN_POINT ( 'NONE',  ( -50.00000000000000000, -70.00000000000000000, 12.49999999999999112 ) ) ;
#26981=ORIENTED_EDGE ( 'NONE', *, *, #16839, .F. ) ;
#26987=ORIENTED_EDGE ( 'NONE', *, *, #18101, .T. ) ;
#26996=ORIENTED_EDGE ( 'NONE', *, *, #20679, .F. ) ;
#27008=ORIENTED_EDGE ( 'NONE', *, *, #9706, .F. ) ;
#27010=PLANE ( 'NONE',  #16069 ) ;
#27023=CARTESIAN_POINT ( 'NONE',  ( -44.99999999999955236, -4.926614671774132148E-13, 77.49999999999998579 ) ) ;
#27026=CARTESIAN_POINT ( 'NONE',  ( 0.000000000000000000, 0.000000000000000000, 57.49999999999999289 ) ) ;
#27041=DIRECTION ( 'NONE',  ( -1.000000000000000000, 0.000000000000000000, 0.000000000000000000 ) ) ;
#27049=EDGE_LOOP ( 'NONE', ( #19629, #3463 ) ) ;
#27083=CARTESIAN_POINT ( 'NONE',  ( 37.16608720827707657, 65.00000000000000000, 97.07879600563551037 ) ) ;
#27085=CARTESIAN_POINT ( 'NONE',  ( -37.16608720827707657, 65.00000000000000000, 12.49999999999999112 ) ) ;
#27088=ORIENTED_EDGE ( 'NONE', *, *, #7646, .F. ) ;
#27090=AXIS2_PLACEMENT_3D ( 'NONE', #9347, #2317, #11844 ) ;
#27097=CIRCLE ( 'NONE', #2190, 3.000000000000002665 ) ;
#27108=ORIENTED_EDGE ( 'NONE', *, *, #27842, .F. ) ;
#27110=ADVANCED_FACE ( 'NONE', ( #4813 ), #23524, .F. ) ;
#27117=CYLINDRICAL_SURFACE ( 'NONE', #9239, 20.00000000000000355 ) ;
#27122=CARTESIAN_POINT ( 'NONE',  ( -40.00000000000000000, 90.00000000000001421, 15.49999999999998934 ) ) ;
#27132=ORIENTED_EDGE ( 'NONE', *, *, #10503, .T. ) ;
#27137=ORIENTED_EDGE ( 'NONE', *, *, #8661, .F. ) ;
#27139=DIRECTION ( 'NONE',  ( -0.000000000000000000, -0.000000000000000000, -1.000000000000000000 ) ) ;
#27152=EDGE_CURVE ( 'NONE', #19059, #16046, #26182, .T. ) ;
#27155=EDGE_CURVE ( 'NONE', #19850, #20585, #4664, .T. ) ;
#27158=FACE_OUTER_BOUND ( 'NONE', #5356, .T. ) ;
#27163=CARTESIAN_POINT ( 'NONE',  ( -50.00000000000000000, 70.00000000000000000, 22.49999999999999289 ) ) ;
#27166=CARTESIAN_POINT ( 'NONE',  ( -40.00000000000002842, 80.00000000000001421, 52.50000000000014921 ) ) ;
#27174=DIRECTION ( 'NONE',  ( -0.000000000000000000, -0.000000000000000000, -1.000000000000000000 ) ) ;
#27181=EDGE_CURVE ( 'NONE', #4505, #28974, #24140, .T. ) ;
#27225=AXIS2_PLACEMENT_3D ( 'NONE', #12537, #17198, #14558 ) ;
#27226=FACE_OUTER_BOUND ( 'NONE', #27790, .T. ) ;
#27235=CYLINDRICAL_SURFACE ( 'NONE', #3891, 34.99999999999933920 ) ;
#27240=DIRECTION ( 'NONE',  ( 1.000000000000000000, -0.000000000000000000, -0.000000000000000000 ) ) ;
#27246=FACE_OUTER_BOUND ( 'NONE', #14887, .T. ) ;
#27249=CIRCLE ( 'NONE', #8335, 2.999999999999999112 ) ;
#27269=DIRECTION ( 'NONE',  ( 0.000000000000000000, 1.000000000000000000, 0.000000000000000000 ) ) ;
#27292=CARTESIAN_POINT ( 'NONE',  ( 0.000000000000000000, 0.000000000000000000, 85.49999999999998579 ) ) ;
#27295=EDGE_CURVE ( 'NONE', #9423, #15798, #13120, .T. ) ;
#27305=AXIS2_PLACEMENT_3D ( 'NONE', #14806, #12789, #2805 ) ;
#27312=VERTEX_POINT ( 'NONE', #24762 ) ;
#27321=ORIENTED_EDGE ( 'NONE', *, *, #12862, .T. ) ;
#27343=EDGE_CURVE ( 'NONE', #12499, #4980, #8564, .T. ) ;
#27348=VERTEX_POINT ( 'NONE', #25693 ) ;
#27349=ADVANCED_FACE ( 'NONE', ( #4321 ), #6661, .F. ) ;
#27355=DIRECTION ( 'NONE',  ( 0.000000000000000000, -1.000000000000000000, 0.000000000000000000 ) ) ;
#27356=CARTESIAN_POINT ( 'NONE',  ( 52.16608720827707657, 51.86186943028246787, 12.49999999999998401 ) ) ;
#27366=EDGE_CURVE ( 'NONE', #353, #17425, #2150, .T. ) ;
#27367=EDGE_CURVE ( 'NONE', #5751, #23685, #17090, .T. ) ;
#27394=PLANE ( 'NONE',  #6838 ) ;
#27401=CYLINDRICAL_SURFACE ( 'NONE', #17269, 20.00000000000000000 ) ;
#27403=DIRECTION ( 'NONE',  ( 0.000000000000000000, 0.000000000000000000, -1.000000000000000000 ) ) ;
#27404=EDGE_CURVE ( 'NONE', #27728, #14860, #28533, .T. ) ;
#27420=CARTESIAN_POINT ( 'NONE',  ( -50.00000000000000000, -50.00000000000000000, 59.49999999999999289 ) ) ;
#27434=LINE ( 'NONE', #24610, #26285 ) ;
#27446=CARTESIAN_POINT ( 'NONE',  ( 49.99999999999998579, 50.00000000000000000, 59.49999999999999289 ) ) ;
#27464=ORIENTED_EDGE ( 'NONE', *, *, #24475, .F. ) ;
#27467=ORIENTED_EDGE ( 'NONE', *, *, #2134, .F. ) ;
#27480=CARTESIAN_POINT ( 'NONE',  ( 64.99999999999998579, 36.86186943028246787, 12.49999999999999112 ) ) ;
#27496=CARTESIAN_POINT ( 'NONE',  ( -37.16608720827707657, 65.00000000000000000, 97.07879600563551037 ) ) ;
#27511=DIRECTION ( 'NONE',  ( 0.000000000000000000, 1.000000000000000000, 0.000000000000000000 ) ) ;
#27512=ORIENTED_EDGE ( 'NONE', *, *, #30347, .F. ) ;
#27520=EDGE_CURVE ( 'NONE', #29034, #20557, #5829, .T. ) ;
#27549=VECTOR ( 'NONE', #26438, 1000.000000000000000 ) ;
#27560=FACE_OUTER_BOUND ( 'NONE', #15523, .T. ) ;
#27563=EDGE_LOOP ( 'NONE', ( #7475, #13890 ) ) ;
#27575=EDGE_LOOP ( 'NONE', ( #13223, #16499, #25335, #21991 ) ) ;
#27581=ORIENTED_EDGE ( 'NONE', *, *, #29770, .F. ) ;
#27600=CARTESIAN_POINT ( 'NONE',  ( 47.15436764833695094, 69.79802288849539593, 15.50528903784843671 ) ) ;
#27603=VERTEX_POINT ( 'NONE', #17376 ) ;
#27614=AXIS2_PLACEMENT_3D ( 'NONE', #17076, #2583, #7573 ) ;
#27615=EDGE_LOOP ( 'NONE', ( #17955, #7052, #392, #2996, #12950 ) ) ;
#27619=FACE_OUTER_BOUND ( 'NONE', #13416, .T. ) ;
#27648=EDGE_CURVE ( 'NONE', #27603, #15359, #997, .T. ) ;
#27668=DIRECTION ( 'NONE',  ( -1.000000000000000000, 0.000000000000000000, 0.000000000000000000 ) ) ;
#27671=EDGE_CURVE ( 'NONE', #6221, #22536, #19585, .T. ) ;
#27679=ORIENTED_EDGE ( 'NONE', *, *, #28020, .F. ) ;
#27716=LINE ( 'NONE', #11183, #4216 ) ;
#27723=AXIS2_PLACEMENT_3D ( 'NONE', #12925, #29292, #10249 ) ;
#27728=VERTEX_POINT ( 'NONE', #29858 ) ;
#27763=CYLINDRICAL_SURFACE ( 'NONE', #5291, 10.00000000000000178 ) ;
#27777=ORIENTED_EDGE ( 'NONE', *, *, #16839, .T. ) ;
#27790=EDGE_LOOP ( 'NONE', ( #8855, #2396, #1160, #6654 ) ) ;
#27792=EDGE_CURVE ( 'NONE', #4577, #25866, #25479, .T. ) ;
#27806=DIRECTION ( 'NONE',  ( 0.000000000000000000, 0.000000000000000000, 1.000000000000000000 ) ) ;
#27819=DIRECTION ( 'NONE',  ( 0.000000000000000000, 0.000000000000000000, -1.000000000000000000 ) ) ;
#27842=EDGE_CURVE ( 'NONE', #10610, #17425, #19152, .T. ) ;
#27844=VECTOR ( 'NONE', #12555, 1000.000000000000000 ) ;
#27850=CARTESIAN_POINT ( 'NONE',  ( 37.99999999999999289, 65.00000000000000000, 15.49999999999998934 ) ) ;
#27856=EDGE_CURVE ( 'NONE', #24053, #16566, #30298, .T. ) ;
#27861=DIRECTION ( 'NONE',  ( -1.000000000000000000, 0.000000000000000000, 0.000000000000000000 ) ) ;
#27887=CARTESIAN_POINT ( 'NONE',  ( -42.49999999999998579, 50.00000000000000000, 12.49999999999999112 ) ) ;
#27896=CARTESIAN_POINT ( 'NONE',  ( 46.99999999999998579, 87.00000000000001421, 22.49999999999999289 ) ) ;
#27903=ORIENTED_EDGE ( 'NONE', *, *, #30413, .T. ) ;
#27908=ORIENTED_EDGE ( 'NONE', *, *, #21350, .T. ) ;
#27909=DIRECTION ( 'NONE',  ( 1.000000000000000000, 0.000000000000000000, 0.000000000000000000 ) ) ;
#27916=PLANE ( 'NONE',  #7301 ) ;
#27928=DIRECTION ( 'NONE',  ( 0.000000000000000000, 1.000000000000000000, -0.000000000000000000 ) ) ;
#27942=DIRECTION ( 'NONE',  ( 1.000000000000000000, 0.000000000000000000, 0.000000000000000000 ) ) ;
#27963=CARTESIAN_POINT ( 'NONE',  ( 49.99999999999998579, 70.00000000000000000, 52.49999999999999289 ) ) ;
#27976=DIRECTION ( 'NONE',  ( 0.000000000000000000, -0.000000000000000000, 1.000000000000000000 ) ) ;
#27986=VERTEX_POINT ( 'NONE', #7044 ) ;
#27995=ORIENTED_EDGE ( 'NONE', *, *, #29759, .T. ) ;
#27999=CARTESIAN_POINT ( 'NONE',  ( -47.15881708134175199, 69.79865606594935912, 15.50986296560572875 ) ) ;
#28001=CARTESIAN_POINT ( 'NONE',  ( 49.99999999999998579, 50.00000000000000000, 97.07879600563551037 ) ) ;
#28004=CARTESIAN_POINT ( 'NONE',  ( 0.000000000000000000, 0.000000000000000000, 85.49999999999998579 ) ) ;
#28020=EDGE_CURVE ( 'NONE', #29733, #20591, #30737, .T. ) ;
#28045=VECTOR ( 'NONE', #3496, 1000.000000000000000 ) ;
#28049=ORIENTED_EDGE ( 'NONE', *, *, #8260, .T. ) ;
#28051=EDGE_CURVE ( 'NONE', #5139, #11277, #10469, .T. ) ;
#28061=EDGE_CURVE ( 'NONE', #24670, #2627, #8138, .T. ) ;
#28065=EDGE_LOOP ( 'NONE', ( #18693, #10913, #23944, #16924 ) ) ;
#28066=ORIENTED_EDGE ( 'NONE', *, *, #3470, .T. ) ;
#28070=AXIS2_PLACEMENT_3D ( 'NONE', #14039, #30571, #28549 ) ;
#28072=CARTESIAN_POINT ( 'NONE',  ( -2.081668171172168513E-14, 75.00000000000001421, 37.49999999999999289 ) ) ;
#28080=FACE_OUTER_BOUND ( 'NONE', #19547, .T. ) ;
#28102=EDGE_CURVE ( 'NONE', #9249, #9573, #4849, .T. ) ;
#28105=CARTESIAN_POINT ( 'NONE',  ( -50.00000000000000000, 50.00000000000000000, 97.07879600563551037 ) ) ;
#28112=CARTESIAN_POINT ( 'NONE',  ( -40.00000000000002842, 80.00000000000001421, 52.50000000000014921 ) ) ;
#28117=DIRECTION ( 'NONE',  ( 0.000000000000000000, 0.000000000000000000, -1.000000000000000000 ) ) ;
#28119=ORIENTED_EDGE ( 'NONE', *, *, #28270, .F. ) ;
#28125=EDGE_CURVE ( 'NONE', #9621, #20672, #15308, .T. ) ;
#28136=ORIENTED_EDGE ( 'NONE', *, *, #18563, .F. ) ;
#28140=CARTESIAN_POINT ( 'NONE',  ( 37.16608720827707657, -65.00000000000000000, 57.49999999999999289 ) ) ;
#28147=DIRECTION ( 'NONE',  ( 0.000000000000000000, 0.000000000000000000, 1.000000000000000000 ) ) ;
#28197=CARTESIAN_POINT ( 'NONE',  ( 46.99999999999998579, 90.00000000000001421, 22.49999999999999289 ) ) ;
#28214=DIRECTION ( 'NONE',  ( 0.000000000000000000, 1.000000000000000000, 0.000000000000000000 ) ) ;
#28231=( GEOMETRIC_REPRESENTATION_CONTEXT ( 3 ) GLOBAL_UNCERTAINTY_ASSIGNED_CONTEXT ( ( #16703 ) ) GLOBAL_UNIT_ASSIGNED_CONTEXT ( ( #9309, #1836, #2133 ) ) REPRESENTATION_CONTEXT ( 'NONE', 'WORKASPACE' ) );
#28238=VECTOR ( 'NONE', #14046, 1000.000000000000000 ) ;
#28270=EDGE_CURVE ( 'NONE', #16046, #14399, #19322, .T. ) ;
#28273=DIRECTION ( 'NONE',  ( -0.000000000000000000, -0.000000000000000000, 1.000000000000000000 ) ) ;
#28302=DIRECTION ( 'NONE',  ( 1.000000000000000000, 0.000000000000000000, 0.000000000000000000 ) ) ;
#28303=VERTEX_POINT ( 'NONE', #25633 ) ;
#28314=LINE ( 'NONE', #22997, #2928 ) ;
#28321=CARTESIAN_POINT ( 'NONE',  ( -38.00000000000000711, 80.00000000000001421, 27.08257569495566841 ) ) ;
#28322=DIRECTION ( 'NONE',  ( 1.000000000000000000, 0.000000000000000000, 0.000000000000000000 ) ) ;
#28325=PLANE ( 'NONE',  #29546 ) ;
#28326=ORIENTED_EDGE ( 'NONE', *, *, #6189, .F. ) ;
#28339=DIRECTION ( 'NONE',  ( 0.000000000000000000, 1.000000000000000000, -0.000000000000000000 ) ) ;
#28358=FACE_OUTER_BOUND ( 'NONE', #26421, .T. ) ;
#28369=ORIENTED_EDGE ( 'NONE', *, *, #9968, .T. ) ;
#28376=ORIENTED_EDGE ( 'NONE', *, *, #28456, .T. ) ;
#28403=EDGE_LOOP ( 'NONE', ( #28494, #146 ) ) ;
#28413=EDGE_LOOP ( 'NONE', ( #21264, #5888 ) ) ;
#28437=DIRECTION ( 'NONE',  ( -1.000000000000000000, 0.000000000000000000, 0.000000000000000000 ) ) ;
#28440=ORIENTED_EDGE ( 'NONE', *, *, #5540, .T. ) ;
#28442=VECTOR ( 'NONE', #8375, 1000.000000000000000 ) ;
#28446=CARTESIAN_POINT ( 'NONE',  ( -50.00000000000000000, 50.00000000000000000, 59.49999999999999289 ) ) ;
#28454=ORIENTED_EDGE ( 'NONE', *, *, #10312, .T. ) ;
#28456=EDGE_CURVE ( 'NONE', #14399, #10610, #22797, .T. ) ;
#28462=DIRECTION ( 'NONE',  ( 0.000000000000000000, 0.000000000000000000, -1.000000000000000000 ) ) ;
#28463=DIRECTION ( 'NONE',  ( -0.000000000000000000, 1.000000000000000000, -0.000000000000000000 ) ) ;
#28470=DIRECTION ( 'NONE',  ( 0.000000000000000000, 0.000000000000000000, -1.000000000000000000 ) ) ;
#28494=ORIENTED_EDGE ( 'NONE', *, *, #10806, .F. ) ;
#28498=EDGE_LOOP ( 'NONE', ( #1423, #20592, #22044, #19176 ) ) ;
#28506=ORIENTED_EDGE ( 'NONE', *, *, #25413, .F. ) ;
#28507=CARTESIAN_POINT ( 'NONE',  ( -42.49999999999998579, 50.00000000000000000, 62.49999999999999289 ) ) ;
#28508=AXIS2_PLACEMENT_3D ( 'NONE', #5359, #17521, #8168 ) ;
#28514=DIRECTION ( 'NONE',  ( 0.000000000000000000, 0.000000000000000000, 1.000000000000000000 ) ) ;
#28533=CIRCLE ( 'NONE', #13619, 17.00000000000000000 ) ;
#28548=DIRECTION ( 'NONE',  ( -1.000000000000000000, 0.000000000000000000, 0.000000000000000000 ) ) ;
#28549=DIRECTION ( 'NONE',  ( -1.000000000000000000, 0.000000000000000000, 0.000000000000000000 ) ) ;
#28559=VERTEX_POINT ( 'NONE', #16382 ) ;
#28566=CARTESIAN_POINT ( 'NONE',  ( 7.483314773547865784, 75.00000000000001421, 50.49999999999998579 ) ) ;
#28568=CARTESIAN_POINT ( 'NONE',  ( 39.99999999999998579, 90.00000000000001421, 57.49999999999998579 ) ) ;
#28570=DIRECTION ( 'NONE',  ( -1.000000000000000000, 0.000000000000000000, 0.000000000000000000 ) ) ;
#28591=VERTEX_POINT ( 'NONE', #24000 ) ;
#28616=DIRECTION ( 'NONE',  ( 0.000000000000000000, 1.000000000000000000, 0.000000000000000000 ) ) ;
#28624=DIRECTION ( 'NONE',  ( 1.000000000000000000, 0.000000000000000000, 0.000000000000000000 ) ) ;
#28625=VERTEX_POINT ( 'NONE', #7022 ) ;
#28632=ORIENTED_EDGE ( 'NONE', *, *, #18143, .F. ) ;
#28668=CARTESIAN_POINT ( 'NONE',  ( 49.99999999999998579, -50.00000000000000000, 97.07879600563551037 ) ) ;
#28691=ORIENTED_EDGE ( 'NONE', *, *, #17924, .F. ) ;
#28694=VECTOR ( 'NONE', #23073, 1000.000000000000000 ) ;
#28717=CARTESIAN_POINT ( 'NONE',  ( 49.99999999999998579, 50.00000000000000000, 12.49999999999999112 ) ) ;
#28722=CARTESIAN_POINT ( 'NONE',  ( 49.37858786280191481, 69.99072022605612631, 55.98525212243750815 ) ) ;
#28725=AXIS2_PLACEMENT_3D ( 'NONE', #6288, #30598, #30451 ) ;
#28730=EDGE_LOOP ( 'NONE', ( #19603, #15500, #21593, #26605 ) ) ;
#28740=CIRCLE ( 'NONE', #20282, 37.99999999999933920 ) ;
#28749=VECTOR ( 'NONE', #25892, 1000.000000000000000 ) ;
#28767=VECTOR ( 'NONE', #28117, 1000.000000000000000 ) ;
#28768=AXIS2_PLACEMENT_3D ( 'NONE', #6486, #8679, #27861 ) ;
#28773=CARTESIAN_POINT ( 'NONE',  ( -70.00000000000000000, 50.00000000000000000, 12.49999999999999112 ) ) ;
#28778=EDGE_LOOP ( 'NONE', ( #23552, #2081, #1415, #12480 ) ) ;
#28786=DIRECTION ( 'NONE',  ( 0.000000000000000000, 0.000000000000000000, -1.000000000000000000 ) ) ;
#28797=EDGE_CURVE ( 'NONE', #25178, #5791, #6976, .T. ) ;
#28806=DIRECTION ( 'NONE',  ( 0.000000000000000000, 0.000000000000000000, -1.000000000000000000 ) ) ;
#28810=CYLINDRICAL_SURFACE ( 'NONE', #12319, 50.00000000000000000 ) ;
#28823=ADVANCED_FACE ( 'NONE', ( #12586 ), #10078, .T. ) ;
#28832=DIRECTION ( 'NONE',  ( 0.000000000000000000, 1.000000000000000000, 0.000000000000000000 ) ) ;
#28844=CARTESIAN_POINT ( 'NONE',  ( 49.99999999999998579, -70.00000000000000000, 12.49999999999999112 ) ) ;
#28856=CARTESIAN_POINT ( 'NONE',  ( 57.49999999999998579, 50.00000000000000000, 12.49999999999999112 ) ) ;
#28885=LINE ( 'NONE', #8286, #1376 ) ;
#28893=DIRECTION ( 'NONE',  ( -0.000000000000000000, 0.000000000000000000, -1.000000000000000000 ) ) ;
#28909=ORIENTED_EDGE ( 'NONE', *, *, #3282, .F. ) ;
#28926=ORIENTED_EDGE ( 'NONE', *, *, #18064, .T. ) ;
#28940=DIRECTION ( 'NONE',  ( -1.000000000000000000, 0.000000000000000000, 0.000000000000000000 ) ) ;
#28949=DIRECTION ( 'NONE',  ( 1.000000000000000000, 0.000000000000000000, 0.000000000000000000 ) ) ;
#28955=ORIENTED_EDGE ( 'NONE', *, *, #27404, .F. ) ;
#28958=DIRECTION ( 'NONE',  ( -0.000000000000000000, -0.000000000000000000, -1.000000000000000000 ) ) ;
#28967=CARTESIAN_POINT ( 'NONE',  ( -70.00000000000000000, -65.00000000000000000, 57.49999999999999289 ) ) ;
#28974=VERTEX_POINT ( 'NONE', #8675 ) ;
#28982=ORIENTED_EDGE ( 'NONE', *, *, #27181, .F. ) ;
#28989=DIRECTION ( 'NONE',  ( -0.000000000000000000, 0.000000000000000000, 1.000000000000000000 ) ) ;
#29001=CARTESIAN_POINT ( 'NONE',  ( -7.483314773547907528, 80.00000000000000000, 50.49999999999998579 ) ) ;
#29003=CARTESIAN_POINT ( 'NONE',  ( -2.081668171172168513E-14, 75.00000000000001421, 52.49999999999999289 ) ) ;
#29004=EDGE_CURVE ( 'NONE', #23685, #24152, #28314, .T. ) ;
#29028=DIRECTION ( 'NONE',  ( 0.000000000000000000, -1.000000000000000000, -0.000000000000000000 ) ) ;
#29034=VERTEX_POINT ( 'NONE', #25354 ) ;
#29035=DIRECTION ( 'NONE',  ( 0.000000000000000000, -0.000000000000000000, 1.000000000000000000 ) ) ;
#29075=VERTEX_POINT ( 'NONE', #25963 ) ;
#29124=ORIENTED_EDGE ( 'NONE', *, *, #15253, .F. ) ;
#29136=DIRECTION ( 'NONE',  ( 0.000000000000000000, -0.000000000000000000, 1.000000000000000000 ) ) ;
#29155=CIRCLE ( 'NONE', #6733, 20.00000000000000355 ) ;
#29176=CARTESIAN_POINT ( 'NONE',  ( 48.71078001599239826, 69.96156514568451712, 57.45356112030430751 ) ) ;
#29181=VECTOR ( 'NONE', #3746, 1000.000000000000000 ) ;
#29185=ORIENTED_EDGE ( 'NONE', *, *, #30731, .T. ) ;
#29192=CARTESIAN_POINT ( 'NONE',  ( 46.99999999999998579, 90.00000000000001421, 22.49999999999999289 ) ) ;
#29193=ADVANCED_FACE ( 'NONE', ( #9889 ), #16594, .F. ) ;
#29195=CYLINDRICAL_SURFACE ( 'NONE', #8300, 34.99999999999933920 ) ;
#29199=EDGE_CURVE ( 'NONE', #25178, #10235, #19839, .T. ) ;
#29224=EDGE_CURVE ( 'NONE', #2852, #7465, #9373, .T. ) ;
#29233=DIRECTION ( 'NONE',  ( -0.000000000000000000, -1.000000000000000000, -0.000000000000000000 ) ) ;
#29241=LINE ( 'NONE', #14889, #3201 ) ;
#29248=LINE ( 'NONE', #19577, #6229 ) ;
#29252=CARTESIAN_POINT ( 'NONE',  ( -49.99999999999955236, -4.926614671774132148E-13, 79.49999999999998579 ) ) ;
#29255=AXIS2_PLACEMENT_3D ( 'NONE', #27446, #8577, #10748 ) ;
#29261=CARTESIAN_POINT ( 'NONE',  ( 39.99999999999998579, 80.00000000000001421, 22.49999999999999289 ) ) ;
#29263=DIRECTION ( 'NONE',  ( 0.000000000000000000, 0.000000000000000000, 1.000000000000000000 ) ) ;
#29269=VECTOR ( 'NONE', #30254, 1000.000000000000000 ) ;
#29278=LINE ( 'NONE', #26792, #25706 ) ;
#29279=VECTOR ( 'NONE', #8565, 1000.000000000000000 ) ;
#29284=CIRCLE ( 'NONE', #18337, 15.00000000000000000 ) ;
#29292=DIRECTION ( 'NONE',  ( -1.000000000000000000, 0.000000000000000000, 0.000000000000000000 ) ) ;
#29303=AXIS2_PLACEMENT_3D ( 'NONE', #6386, #4038, #13564 ) ;
#29326=CARTESIAN_POINT ( 'NONE',  ( -4.163336342344337027E-14, 1.387778780781445676E-14, 67.49999999999997158 ) ) ;
#29329=ORIENTED_EDGE ( 'NONE', *, *, #23445, .T. ) ;
#29334=ORIENTED_EDGE ( 'NONE', *, *, #16097, .F. ) ;
#29335=LINE ( 'NONE', #8125, #18807 ) ;
#29348=CARTESIAN_POINT ( 'NONE',  ( -7.075845757273814415E-16, 80.00000000000000000, 15.49999999999998757 ) ) ;
#29356=AXIS2_PLACEMENT_3D ( 'NONE', #21753, #22219, #854 ) ;
#29360=CARTESIAN_POINT ( 'NONE',  ( -40.00000000000000000, 63.74772708486752038, 62.49999999999999289 ) ) ;
#29383=DIRECTION ( 'NONE',  ( -0.000000000000000000, 1.000000000000000000, -0.000000000000000000 ) ) ;
#29410=EDGE_CURVE ( 'NONE', #12825, #30078, #2433, .T. ) ;
#29414=EDGE_CURVE ( 'NONE', #23905, #28303, #11344, .T. ) ;
#29415=CARTESIAN_POINT ( 'NONE',  ( 29.99999999999925038, 1.387778780781445676E-14, 67.49999999999997158 ) ) ;
#29428=CARTESIAN_POINT ( 'NONE',  ( -57.50000000000001421, 50.00000000000000000, 12.49999999999999112 ) ) ;
#29434=ORIENTED_EDGE ( 'NONE', *, *, #12994, .F. ) ;
#29447=ORIENTED_EDGE ( 'NONE', *, *, #26444, .T. ) ;
#29456=ORIENTED_EDGE ( 'NONE', *, *, #22521, .F. ) ;
#29481=FACE_OUTER_BOUND ( 'NONE', #11815, .T. ) ;
#29489=ORIENTED_EDGE ( 'NONE', *, *, #3298, .F. ) ;
#29495=ORIENTED_EDGE ( 'NONE', *, *, #27404, .T. ) ;
#29497=CYLINDRICAL_SURFACE ( 'NONE', #22610, 3.000000000000002665 ) ;
#29508=DIRECTION ( 'NONE',  ( -0.000000000000000000, -0.000000000000000000, -1.000000000000000000 ) ) ;
#29512=CARTESIAN_POINT ( 'NONE',  ( -46.52886832597424416, 69.65281066659318299, 60.08552421216484873 ) ) ;
#29515=DIRECTION ( 'NONE',  ( 0.000000000000000000, -1.000000000000000000, 0.000000000000000000 ) ) ;
#29518=CARTESIAN_POINT ( 'NONE',  ( 14.99999999999995737, 1.387778780781445676E-14, 77.49999999999998579 ) ) ;
#29529=ORIENTED_EDGE ( 'NONE', *, *, #27520, .T. ) ;
#29546=AXIS2_PLACEMENT_3D ( 'NONE', #4290, #9131, #18651 ) ;
#29567=AXIS2_PLACEMENT_3D ( 'NONE', #24941, #3579, #27909 ) ;
#29568=CIRCLE ( 'NONE', #8157, 4.999999999999997335 ) ;
#29570=DIRECTION ( 'NONE',  ( 1.000000000000000000, 0.000000000000000000, 0.000000000000000000 ) ) ;
#29583=EDGE_CURVE ( 'NONE', #22741, #10498, #17644, .T. ) ;
#29601=DIRECTION ( 'NONE',  ( 0.000000000000000000, 0.000000000000000000, -1.000000000000000000 ) ) ;
#29607=AXIS2_PLACEMENT_3D ( 'NONE', #29326, #21983, #5464 ) ;
#29609=DIRECTION ( 'NONE',  ( 1.000000000000000000, 0.000000000000000000, 0.000000000000000000 ) ) ;
#29619=FACE_OUTER_BOUND ( 'NONE', #23955, .T. ) ;
#29620=ADVANCED_FACE ( 'NONE', ( #14878 ), #16751, .T. ) ;
#29626=CARTESIAN_POINT ( 'NONE',  ( -37.16608720827707657, 65.00000000000000000, 97.07879600563551037 ) ) ;
#29639=VERTEX_POINT ( 'NONE', #26432 ) ;
#29662=CARTESIAN_POINT ( 'NONE',  ( -44.92384265402849763, 68.80442260972010615, 61.21192266590395548 ) ) ;
#29667=FACE_BOUND ( 'NONE', #20129, .T. ) ;
#29682=LINE ( 'NONE', #18459, #6535 ) ;
#29685=VECTOR ( 'NONE', #27511, 1000.000000000000000 ) ;
#29690=ORIENTED_EDGE ( 'NONE', *, *, #12460, .T. ) ;
#29701=LINE ( 'NONE', #8345, #3450 ) ;
#29721=ORIENTED_EDGE ( 'NONE', *, *, #30413, .F. ) ;
#29733=VERTEX_POINT ( 'NONE', #219 ) ;
#29739=AXIS2_PLACEMENT_3D ( 'NONE', #12193, #330, #26394 ) ;
#29741=( NAMED_UNIT ( * ) PLANE_ANGLE_UNIT ( ) SI_UNIT ( $, .RADIAN. ) );
#29746=ORIENTED_EDGE ( 'NONE', *, *, #1524, .T. ) ;
#29756=EDGE_CURVE ( 'NONE', #22640, #29034, #682, .T. ) ;
#29758=CIRCLE ( 'NONE', #16620, 15.00000000000000000 ) ;
#29759=EDGE_CURVE ( 'NONE', #10854, #977, #15884, .T. ) ;
#29770=EDGE_CURVE ( 'NONE', #12261, #28625, #19782, .T. ) ;
#29777=VECTOR ( 'NONE', #12363, 1000.000000000000000 ) ;
#29803=ORIENTED_EDGE ( 'NONE', *, *, #20958, .T. ) ;
#29804=AXIS2_PLACEMENT_3D ( 'NONE', #9516, #19034, #28548 ) ;
#29808=DIRECTION ( 'NONE',  ( 0.000000000000000000, 0.000000000000000000, 1.000000000000000000 ) ) ;
#29809=ORIENTED_EDGE ( 'NONE', *, *, #22521, .T. ) ;
#29815=LINE ( 'NONE', #1714, #29269 ) ;
#29825=ORIENTED_EDGE ( 'NONE', *, *, #6743, .T. ) ;
#29832=DIRECTION ( 'NONE',  ( -0.000000000000000000, -0.000000000000000000, 1.000000000000000000 ) ) ;
#29834=EDGE_CURVE ( 'NONE', #7465, #25448, #16808, .T. ) ;
#29836=VECTOR ( 'NONE', #26011, 1000.000000000000000 ) ;
#29842=AXIS2_PLACEMENT_3D ( 'NONE', #17794, #19974, #29808 ) ;
#29850=DIRECTION ( 'NONE',  ( -0.000000000000000000, -0.000000000000000000, 1.000000000000000000 ) ) ;
#29858=CARTESIAN_POINT ( 'NONE',  ( -40.00000000000000000, 63.74772708486752038, 62.49999999999999289 ) ) ;
#29859=LINE ( 'NONE', #8499, #26178 ) ;
#29881=ORIENTED_EDGE ( 'NONE', *, *, #10143, .F. ) ;
#29888=VECTOR ( 'NONE', #13372, 1000.000000000000000 ) ;
#29901=CIRCLE ( 'NONE', #24923, 34.99999999999933920 ) ;
#29918=EDGE_LOOP ( 'NONE', ( #7528, #15193 ) ) ;
#29921=CARTESIAN_POINT ( 'NONE',  ( 52.16608720827707657, 36.86186943028246787, 12.49999999999999112 ) ) ;
#29959=DIRECTION ( 'NONE',  ( 0.000000000000000000, 0.000000000000000000, 1.000000000000000000 ) ) ;
#29964=EDGE_CURVE ( 'NONE', #15180, #4126, #23300, .T. ) ;
#29975=EDGE_CURVE ( 'NONE', #20802, #16462, #5880, .T. ) ;
#29984=CIRCLE ( 'NONE', #20507, 4.999999999999997335 ) ;
#29991=PLANE ( 'NONE',  #21733 ) ;
#29995=LINE ( 'NONE', #13313, #22732 ) ;
#30013=CARTESIAN_POINT ( 'NONE',  ( 49.99999999999998579, 87.00000000000001421, 52.49999999999999289 ) ) ;
#30036=CARTESIAN_POINT ( 'NONE',  ( -45.91542376395022984, 69.58700628869918603, 14.40979685689198675 ) ) ;
#30042=CARTESIAN_POINT ( 'NONE',  ( -52.16608720827707657, -51.86186943028246787, 12.49999999999998401 ) ) ;
#30052=AXIS2_PLACEMENT_3D ( 'NONE', #10749, #15578, #3739 ) ;
#30070=LINE ( 'NONE', #1838, #3334 ) ;
#30073=B_SPLINE_CURVE_WITH_KNOTS ( 'NONE', 3,
 ( #6384, #13419, #20417, #6067, #11059, #3578, #20559, #8424, #3894, #13255, #25247, #13099, #3738, #27600, #1548, #15575, #22901, #18233, #15418, #1243, #22743, #30084, #1403, #8719 ),
 .UNSPECIFIED., .F., .F.,
 ( 4, 2, 2, 2, 2, 2, 2, 2, 2, 2, 2, 4 ),
 ( 0.000000000000000000, 0.002009995092672920650, 0.003014992639009388999, 0.004019990185345856913, 0.006029985278018779732, 0.007034982824355240708, 0.008039980370691701683, 0.009044977917028164394, 0.01004997546336462363, 0.01205997055603754732, 0.01406996564871046927, 0.01607996074138339296 ),
 .UNSPECIFIED. ) ;
#30078=VERTEX_POINT ( 'NONE', #29415 ) ;
#30084=CARTESIAN_POINT ( 'NONE',  ( 49.93149649555489589, 70.00033699790037645, 21.15209104779357574 ) ) ;
#30098=EDGE_LOOP ( 'NONE', ( #29185, #15466 ) ) ;
#30116=ORIENTED_EDGE ( 'NONE', *, *, #18796, .F. ) ;
#30132=EDGE_CURVE ( 'NONE', #30406, #22536, #1024, .T. ) ;
#30133=ORIENTED_EDGE ( 'NONE', *, *, #16209, .F. ) ;
#30139=ADVANCED_FACE ( 'NONE', ( #5242 ), #10219, .F. ) ;
#30145=CARTESIAN_POINT ( 'NONE',  ( 37.16608720827707657, -65.00000000000000000, 12.49999999999999112 ) ) ;
#30149=EDGE_CURVE ( 'NONE', #8380, #17431, #29284, .T. ) ;
#30184=EDGE_CURVE ( 'NONE', #19467, #22374, #22527, .T. ) ;
#30186=AXIS2_PLACEMENT_3D ( 'NONE', #19523, #29035, #12517 ) ;
#30204=DIRECTION ( 'NONE',  ( 1.000000000000000000, 0.000000000000000000, 0.000000000000000000 ) ) ;
#30205=CIRCLE ( 'NONE', #23701, 7.500000000000013323 ) ;
#30228=ORIENTED_EDGE ( 'NONE', *, *, #4646, .T. ) ;
#30254=DIRECTION ( 'NONE',  ( 0.000000000000000000, 0.000000000000000000, -1.000000000000000000 ) ) ;
#30273=DIRECTION ( 'NONE',  ( 0.000000000000000000, -1.000000000000000000, 0.000000000000000000 ) ) ;
#30289=AXIS2_PLACEMENT_3D ( 'NONE', #8701, #20540, #18827 ) ;
#30295=DIRECTION ( 'NONE',  ( -1.000000000000000000, 0.000000000000000000, 0.000000000000000000 ) ) ;
#30298=LINE ( 'NONE', #13632, #12840 ) ;
#30309=PLANE ( 'NONE',  #13623 ) ;
#30324=VECTOR ( 'NONE', #10622, 1000.000000000000000 ) ;
#30338=CARTESIAN_POINT ( 'NONE',  ( 39.99999999999998579, 87.00000000000001421, 52.49999999999999289 ) ) ;
#30345=DIRECTION ( 'NONE',  ( 0.000000000000000000, 0.000000000000000000, 1.000000000000000000 ) ) ;
#30347=EDGE_CURVE ( 'NONE', #23472, #23537, #24189, .T. ) ;
#30370=LINE ( 'NONE', #1528, #23436 ) ;
#30372=CARTESIAN_POINT ( 'NONE',  ( -40.00000000000002842, 80.00000000000001421, 52.50000000000014921 ) ) ;
#30400=ORIENTED_EDGE ( 'NONE', *, *, #18143, .T. ) ;
#30406=VERTEX_POINT ( 'NONE', #27023 ) ;
#30407=DIRECTION ( 'NONE',  ( 0.000000000000000000, 1.000000000000000000, 0.000000000000000000 ) ) ;
#30408=ORIENTED_EDGE ( 'NONE', *, *, #27295, .F. ) ;
#30413=EDGE_CURVE ( 'NONE', #25485, #18996, #23785, .T. ) ;
#30435=VERTEX_POINT ( 'NONE', #13742 ) ;
#30436=CARTESIAN_POINT ( 'NONE',  ( -37.16608720827707657, -65.00000000000000000, 97.07879600563551037 ) ) ;
#30442=DIRECTION ( 'NONE',  ( -1.000000000000000000, 0.000000000000000000, 0.000000000000000000 ) ) ;
#30451=DIRECTION ( 'NONE',  ( -1.000000000000000000, 0.000000000000000000, 0.000000000000000000 ) ) ;
#30457=EDGE_LOOP ( 'NONE', ( #8714, #29529, #7078, #28691, #1771, #12785 ) ) ;
#30459=FACE_OUTER_BOUND ( 'NONE', #16042, .T. ) ;
#30465=DIRECTION ( 'NONE',  ( -1.000000000000000000, 0.000000000000000000, 0.000000000000000000 ) ) ;
#30471=AXIS2_PLACEMENT_3D ( 'NONE', #1030, #20046, #10539 ) ;
#30492=ORIENTED_EDGE ( 'NONE', *, *, #18362, .F. ) ;
#30495=DIRECTION ( 'NONE',  ( -1.000000000000000000, -1.224646799147308341E-16, 0.000000000000000000 ) ) ;
#30496=VERTEX_POINT ( 'NONE', #30718 ) ;
#30500=ORIENTED_EDGE ( 'NONE', *, *, #10484, .T. ) ;
#30509=ADVANCED_FACE ( 'NONE', ( #4528 ), #26050, .T. ) ;
#30518=CARTESIAN_POINT ( 'NONE',  ( 39.99999999999998579, 87.00000000000001421, 15.49999999999999289 ) ) ;
#30523=DIRECTION ( 'NONE',  ( -0.000000000000000000, -0.000000000000000000, 1.000000000000000000 ) ) ;
#30535=DIRECTION ( 'NONE',  ( 1.224646799147353207E-16, 1.000000000000000000, -0.000000000000000000 ) ) ;
#30546=EDGE_CURVE ( 'NONE', #25524, #4513, #17341, .T. ) ;
#30550=ORIENTED_EDGE ( 'NONE', *, *, #25180, .F. ) ;
#30551=EDGE_CURVE ( 'NONE', #977, #29639, #30781, .T. ) ;
#30571=DIRECTION ( 'NONE',  ( 0.000000000000000000, 0.000000000000000000, -1.000000000000000000 ) ) ;
#30573=AXIS2_PLACEMENT_3D ( 'NONE', #4719, #28437, #18619 ) ;
#30598=DIRECTION ( 'NONE',  ( 0.000000000000000000, 0.000000000000000000, -1.000000000000000000 ) ) ;
#30613=EDGE_LOOP ( 'NONE', ( #21187, #26882, #2600, #22604, #12531, #22408, #30400, #12187, #26418, #16585, #15863, #30500 ) ) ;
#30620=VECTOR ( 'NONE', #2550, 1000.000000000000000 ) ;
#30629=CARTESIAN_POINT ( 'NONE',  ( -40.00000000000000000, 67.32050807568877815, 12.49999999999999112 ) ) ;
#30645=MECHANICAL_DESIGN_GEOMETRIC_PRESENTATION_REPRESENTATION('',(#9803),#28231);
#30650=CARTESIAN_POINT ( 'NONE',  ( -50.00000000000000000, 50.00000000000000000, 12.49999999999999112 ) ) ;
#30653=FACE_OUTER_BOUND ( 'NONE', #21104, .T. ) ;
#30654=CIRCLE ( 'NONE', #23674, 4.999999999999997335 ) ;
#30663=DIRECTION ( 'NONE',  ( -0.000000000000000000, 1.000000000000000000, -0.000000000000000000 ) ) ;
#30677=CARTESIAN_POINT ( 'NONE',  ( -47.14142842854255377, 69.79466010243307039, 59.50000000000029843 ) ) ;
#30678=CIRCLE ( 'NONE', #21207, 3.000000000000002665 ) ;
#30695=AXIS2_PLACEMENT_3D ( 'NONE', #18142, #27355, #6277 ) ;
#30708=AXIS2_PLACEMENT_3D ( 'NONE', #17683, #22505, #13015 ) ;
#30713=AXIS2_PLACEMENT_3D ( 'NONE', #12933, #27269, #8093 ) ;
#30718=CARTESIAN_POINT ( 'NONE',  ( -52.16608720827707657, 36.86186943028246787, 12.49999999999999112 ) ) ;
#30721=AXIS2_PLACEMENT_3D ( 'NONE', #14204, #7518, #325 ) ;
#30731=EDGE_CURVE ( 'NONE', #29639, #22904, #18844, .T. ) ;
#30732=VERTEX_POINT ( 'NONE', #23046 ) ;
#30737=CIRCLE ( 'NONE', #21266, 50.00000000000000000 ) ;
#30747=AXIS2_PLACEMENT_3D ( 'NONE', #22424, #3403, #13235 ) ;
#30781=CIRCLE ( 'NONE', #27305, 3.000000000000002665 ) ;
#30784=DIRECTION ( 'NONE',  ( 1.000000000000000000, 0.000000000000000000, 0.000000000000000000 ) ) ;
#30793=ADVANCED_FACE ( 'NONE', ( #7299 ), #16354, .F. ) ;
#30797=LINE ( 'NONE', #25667, #21975 ) ;
#30800=PLANE ( 'NONE',  #6141 ) ;
#30802=ORIENTED_EDGE ( 'NONE', *, *, #25632, .T. ) ;
#30833=LINE ( 'NONE', #11810, #22357 ) ;
#30837=DIRECTION ( 'NONE',  ( 0.000000000000000000, 0.000000000000000000, -1.000000000000000000 ) ) ;
#30840=DIRECTION ( 'NONE',  ( -1.000000000000000000, 1.224646799147351975E-16, 0.000000000000000000 ) ) ;
#30851=ORIENTED_EDGE ( 'NONE', *, *, #29199, .F. ) ;
#30873=COLOUR_RGB('Dark Blue',0.08,0.2,0.34);
#30874=FILL_AREA_STYLE_COLOUR('',#30873);
#30875=FILL_AREA_STYLE('',(#30874));
#30876=SURFACE_STYLE_FILL_AREA(#30875);
#30877=SURFACE_SIDE_STYLE('',(#30876));
#30878=SURFACE_STYLE_USAGE(.BOTH.,#30877);
#30879=PRESENTATION_STYLE_ASSIGNMENT((#30878));
ENDSEC;
END-ISO-10303-21;
